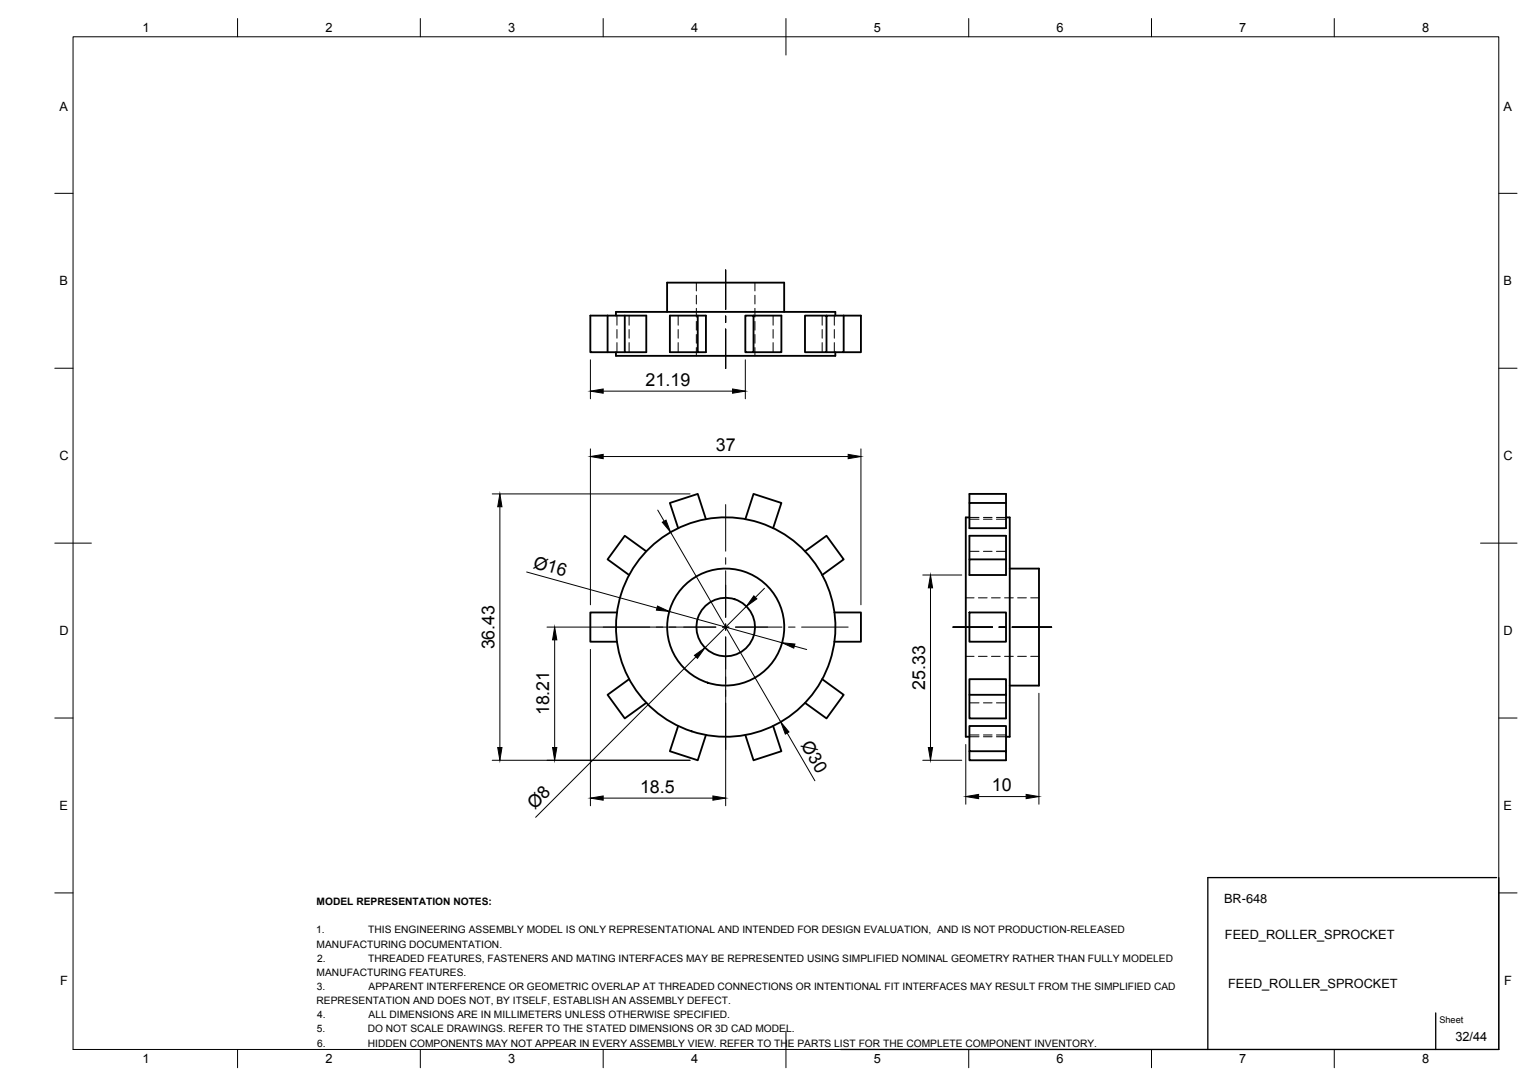
ISO-10303-21;
HEADER;
FILE_DESCRIPTION((''),'2;1');
FILE_NAME('FEED_ROLLER_SPROCKET.step','2026-10-01T22:05:39-07:00',(''),(''),'','','');
FILE_SCHEMA (('AUTOMOTIVE_DESIGN { 1 0 10303 214 3 1 1 }'));
ENDSEC;
DATA;
#10=MECHANICAL_DESIGN_GEOMETRIC_PRESENTATION_REPRESENTATION('',(#630),#24628);
#546=SHAPE_REPRESENTATION_RELATIONSHIP('SRR','None',#24819,#588) ;
#588=ADVANCED_BREP_SHAPE_REPRESENTATION('',(#669),#24609) ;
#630=STYLED_ITEM('',(#25030),#669) ;
#669=MANIFOLD_SOLID_BREP('FEED_ROLLER_SPROCKET',#13172) ;
#888=FACE_BOUND('',#4502,.T.) ;
#889=FACE_BOUND('',#4554,.T.) ;
#890=FACE_BOUND('',#4555,.T.) ;
#891=FACE_BOUND('',#4556,.T.) ;
#892=FACE_BOUND('',#4557,.T.) ;
#893=FACE_BOUND('',#4558,.T.) ;
#894=FACE_BOUND('',#4559,.T.) ;
#895=FACE_BOUND('',#4560,.T.) ;
#896=FACE_BOUND('',#4561,.T.) ;
#897=FACE_BOUND('',#4562,.T.) ;
#898=FACE_BOUND('',#4564,.T.) ;
#899=FACE_BOUND('',#4566,.T.) ;
#1562=LINE('',#23310,#2398) ;
#1563=LINE('',#23316,#2399) ;
#1564=LINE('',#23324,#2400) ;
#1565=LINE('',#23326,#2401) ;
#1566=LINE('',#23327,#2402) ;
#1567=LINE('',#23330,#2403) ;
#1568=LINE('',#23332,#2404) ;
#1569=LINE('',#23333,#2405) ;
#1570=LINE('',#23336,#2406) ;
#1571=LINE('',#23338,#2407) ;
#1572=LINE('',#23339,#2408) ;
#1573=LINE('',#23342,#2409) ;
#1574=LINE('',#23349,#2410) ;
#1575=LINE('',#23351,#2411) ;
#1576=LINE('',#23352,#2412) ;
#1577=LINE('',#23355,#2413) ;
#1578=LINE('',#23357,#2414) ;
#1579=LINE('',#23358,#2415) ;
#1580=LINE('',#23361,#2416) ;
#1581=LINE('',#23363,#2417) ;
#1582=LINE('',#23364,#2418) ;
#1583=LINE('',#23367,#2419) ;
#1584=LINE('',#23374,#2420) ;
#1585=LINE('',#23376,#2421) ;
#1586=LINE('',#23377,#2422) ;
#1587=LINE('',#23380,#2423) ;
#1588=LINE('',#23382,#2424) ;
#1589=LINE('',#23383,#2425) ;
#1590=LINE('',#23386,#2426) ;
#1591=LINE('',#23388,#2427) ;
#1592=LINE('',#23389,#2428) ;
#1593=LINE('',#23392,#2429) ;
#1594=LINE('',#23399,#2430) ;
#1595=LINE('',#23401,#2431) ;
#1596=LINE('',#23402,#2432) ;
#1597=LINE('',#23405,#2433) ;
#1598=LINE('',#23407,#2434) ;
#1599=LINE('',#23408,#2435) ;
#1600=LINE('',#23411,#2436) ;
#1601=LINE('',#23413,#2437) ;
#1602=LINE('',#23414,#2438) ;
#1603=LINE('',#23417,#2439) ;
#1604=LINE('',#23424,#2440) ;
#1605=LINE('',#23426,#2441) ;
#1606=LINE('',#23428,#2442) ;
#1607=LINE('',#23432,#2443) ;
#1608=LINE('',#23434,#2444) ;
#1609=LINE('',#23435,#2445) ;
#1610=LINE('',#23438,#2446) ;
#1611=LINE('',#23440,#2447) ;
#1612=LINE('',#23441,#2448) ;
#1613=LINE('',#23445,#2449) ;
#1614=LINE('',#23453,#2450) ;
#1615=LINE('',#23455,#2451) ;
#1616=LINE('',#23456,#2452) ;
#1617=LINE('',#23459,#2453) ;
#1618=LINE('',#23461,#2454) ;
#1619=LINE('',#23462,#2455) ;
#1620=LINE('',#23465,#2456) ;
#1621=LINE('',#23467,#2457) ;
#1622=LINE('',#23468,#2458) ;
#1623=LINE('',#23471,#2459) ;
#1624=LINE('',#23478,#2460) ;
#1625=LINE('',#23480,#2461) ;
#1626=LINE('',#23481,#2462) ;
#1627=LINE('',#23484,#2463) ;
#1628=LINE('',#23486,#2464) ;
#1629=LINE('',#23487,#2465) ;
#1630=LINE('',#23490,#2466) ;
#1631=LINE('',#23492,#2467) ;
#1632=LINE('',#23493,#2468) ;
#1633=LINE('',#23496,#2469) ;
#1634=LINE('',#23503,#2470) ;
#1635=LINE('',#23505,#2471) ;
#1636=LINE('',#23506,#2472) ;
#1637=LINE('',#23509,#2473) ;
#1638=LINE('',#23511,#2474) ;
#1639=LINE('',#23512,#2475) ;
#1640=LINE('',#23515,#2476) ;
#1641=LINE('',#23517,#2477) ;
#1642=LINE('',#23518,#2478) ;
#1643=LINE('',#23521,#2479) ;
#1644=LINE('',#23528,#2480) ;
#1645=LINE('',#23530,#2481) ;
#1646=LINE('',#23531,#2482) ;
#1647=LINE('',#23534,#2483) ;
#1648=LINE('',#23536,#2484) ;
#1649=LINE('',#23537,#2485) ;
#1650=LINE('',#23540,#2486) ;
#1651=LINE('',#23542,#2487) ;
#1652=LINE('',#23543,#2488) ;
#1653=LINE('',#23546,#2489) ;
#1654=LINE('',#23553,#2490) ;
#1655=LINE('',#23555,#2491) ;
#1656=LINE('',#23556,#2492) ;
#1657=LINE('',#23559,#2493) ;
#1658=LINE('',#23561,#2494) ;
#1659=LINE('',#23562,#2495) ;
#1660=LINE('',#23565,#2496) ;
#1661=LINE('',#23567,#2497) ;
#1662=LINE('',#23568,#2498) ;
#1663=LINE('',#23571,#2499) ;
#1664=LINE('',#23576,#2500) ;
#1665=LINE('',#23578,#2501) ;
#2398=VECTOR('',#18669,0.4) ;
#2399=VECTOR('',#18676,0.8) ;
#2400=VECTOR('',#18685,1.) ;
#2401=VECTOR('',#18686,1.) ;
#2402=VECTOR('',#18687,1.) ;
#2403=VECTOR('',#18690,1.) ;
#2404=VECTOR('',#18691,1.) ;
#2405=VECTOR('',#18692,1.) ;
#2406=VECTOR('',#18695,1.) ;
#2407=VECTOR('',#18696,1.) ;
#2408=VECTOR('',#18697,1.) ;
#2409=VECTOR('',#18702,1.) ;
#2410=VECTOR('',#18709,1.) ;
#2411=VECTOR('',#18710,1.) ;
#2412=VECTOR('',#18711,1.) ;
#2413=VECTOR('',#18714,1.) ;
#2414=VECTOR('',#18715,1.) ;
#2415=VECTOR('',#18716,1.) ;
#2416=VECTOR('',#18719,1.) ;
#2417=VECTOR('',#18720,1.) ;
#2418=VECTOR('',#18721,1.) ;
#2419=VECTOR('',#18726,1.) ;
#2420=VECTOR('',#18733,1.) ;
#2421=VECTOR('',#18734,1.) ;
#2422=VECTOR('',#18735,1.) ;
#2423=VECTOR('',#18738,1.) ;
#2424=VECTOR('',#18739,1.) ;
#2425=VECTOR('',#18740,1.) ;
#2426=VECTOR('',#18743,1.) ;
#2427=VECTOR('',#18744,1.) ;
#2428=VECTOR('',#18745,1.) ;
#2429=VECTOR('',#18750,1.) ;
#2430=VECTOR('',#18757,1.) ;
#2431=VECTOR('',#18758,1.) ;
#2432=VECTOR('',#18759,1.) ;
#2433=VECTOR('',#18762,1.) ;
#2434=VECTOR('',#18763,1.) ;
#2435=VECTOR('',#18764,1.) ;
#2436=VECTOR('',#18767,1.) ;
#2437=VECTOR('',#18768,1.) ;
#2438=VECTOR('',#18769,1.) ;
#2439=VECTOR('',#18774,1.) ;
#2440=VECTOR('',#18781,1.) ;
#2441=VECTOR('',#18782,1.) ;
#2442=VECTOR('',#18783,1.) ;
#2443=VECTOR('',#18788,1.) ;
#2444=VECTOR('',#18789,1.) ;
#2445=VECTOR('',#18790,1.) ;
#2446=VECTOR('',#18793,1.) ;
#2447=VECTOR('',#18794,1.) ;
#2448=VECTOR('',#18795,1.) ;
#2449=VECTOR('',#18800,1.) ;
#2450=VECTOR('',#18809,1.) ;
#2451=VECTOR('',#18810,1.) ;
#2452=VECTOR('',#18811,1.) ;
#2453=VECTOR('',#18814,1.) ;
#2454=VECTOR('',#18815,1.) ;
#2455=VECTOR('',#18816,1.) ;
#2456=VECTOR('',#18819,1.) ;
#2457=VECTOR('',#18820,1.) ;
#2458=VECTOR('',#18821,1.) ;
#2459=VECTOR('',#18826,1.) ;
#2460=VECTOR('',#18833,1.) ;
#2461=VECTOR('',#18834,1.) ;
#2462=VECTOR('',#18835,1.) ;
#2463=VECTOR('',#18838,1.) ;
#2464=VECTOR('',#18839,1.) ;
#2465=VECTOR('',#18840,1.) ;
#2466=VECTOR('',#18843,1.) ;
#2467=VECTOR('',#18844,1.) ;
#2468=VECTOR('',#18845,1.) ;
#2469=VECTOR('',#18850,1.) ;
#2470=VECTOR('',#18857,1.) ;
#2471=VECTOR('',#18858,1.) ;
#2472=VECTOR('',#18859,1.) ;
#2473=VECTOR('',#18862,1.) ;
#2474=VECTOR('',#18863,1.) ;
#2475=VECTOR('',#18864,1.) ;
#2476=VECTOR('',#18867,1.) ;
#2477=VECTOR('',#18868,1.) ;
#2478=VECTOR('',#18869,1.) ;
#2479=VECTOR('',#18874,1.) ;
#2480=VECTOR('',#18881,1.) ;
#2481=VECTOR('',#18882,1.) ;
#2482=VECTOR('',#18883,1.) ;
#2483=VECTOR('',#18886,1.) ;
#2484=VECTOR('',#18887,1.) ;
#2485=VECTOR('',#18888,1.) ;
#2486=VECTOR('',#18891,1.) ;
#2487=VECTOR('',#18892,1.) ;
#2488=VECTOR('',#18893,1.) ;
#2489=VECTOR('',#18898,1.) ;
#2490=VECTOR('',#18905,1.) ;
#2491=VECTOR('',#18906,1.) ;
#2492=VECTOR('',#18907,1.) ;
#2493=VECTOR('',#18910,1.) ;
#2494=VECTOR('',#18911,1.) ;
#2495=VECTOR('',#18912,1.) ;
#2496=VECTOR('',#18915,1.) ;
#2497=VECTOR('',#18916,1.) ;
#2498=VECTOR('',#18917,1.) ;
#2499=VECTOR('',#18922,1.) ;
#2500=VECTOR('',#18929,1.5) ;
#2501=VECTOR('',#18930,1.5) ;
#2900=CYLINDRICAL_SURFACE('',#15009,0.4) ;
#2901=CYLINDRICAL_SURFACE('',#15012,0.8) ;
#2902=CYLINDRICAL_SURFACE('',#15088,1.5) ;
#3530=FACE_OUTER_BOUND('',#4499,.T.) ;
#3531=FACE_OUTER_BOUND('',#4500,.T.) ;
#3532=FACE_OUTER_BOUND('',#4501,.T.) ;
#3533=FACE_OUTER_BOUND('',#4503,.T.) ;
#3534=FACE_OUTER_BOUND('',#4504,.T.) ;
#3535=FACE_OUTER_BOUND('',#4505,.T.) ;
#3536=FACE_OUTER_BOUND('',#4506,.T.) ;
#3537=FACE_OUTER_BOUND('',#4507,.T.) ;
#3538=FACE_OUTER_BOUND('',#4508,.T.) ;
#3539=FACE_OUTER_BOUND('',#4509,.T.) ;
#3540=FACE_OUTER_BOUND('',#4510,.T.) ;
#3541=FACE_OUTER_BOUND('',#4511,.T.) ;
#3542=FACE_OUTER_BOUND('',#4512,.T.) ;
#3543=FACE_OUTER_BOUND('',#4513,.T.) ;
#3544=FACE_OUTER_BOUND('',#4514,.T.) ;
#3545=FACE_OUTER_BOUND('',#4515,.T.) ;
#3546=FACE_OUTER_BOUND('',#4516,.T.) ;
#3547=FACE_OUTER_BOUND('',#4517,.T.) ;
#3548=FACE_OUTER_BOUND('',#4518,.T.) ;
#3549=FACE_OUTER_BOUND('',#4519,.T.) ;
#3550=FACE_OUTER_BOUND('',#4520,.T.) ;
#3551=FACE_OUTER_BOUND('',#4521,.T.) ;
#3552=FACE_OUTER_BOUND('',#4522,.T.) ;
#3553=FACE_OUTER_BOUND('',#4523,.T.) ;
#3554=FACE_OUTER_BOUND('',#4524,.T.) ;
#3555=FACE_OUTER_BOUND('',#4525,.T.) ;
#3556=FACE_OUTER_BOUND('',#4526,.T.) ;
#3557=FACE_OUTER_BOUND('',#4527,.T.) ;
#3558=FACE_OUTER_BOUND('',#4528,.T.) ;
#3559=FACE_OUTER_BOUND('',#4529,.T.) ;
#3560=FACE_OUTER_BOUND('',#4530,.T.) ;
#3561=FACE_OUTER_BOUND('',#4531,.T.) ;
#3562=FACE_OUTER_BOUND('',#4532,.T.) ;
#3563=FACE_OUTER_BOUND('',#4533,.T.) ;
#3564=FACE_OUTER_BOUND('',#4534,.T.) ;
#3565=FACE_OUTER_BOUND('',#4535,.T.) ;
#3566=FACE_OUTER_BOUND('',#4536,.T.) ;
#3567=FACE_OUTER_BOUND('',#4537,.T.) ;
#3568=FACE_OUTER_BOUND('',#4538,.T.) ;
#3569=FACE_OUTER_BOUND('',#4539,.T.) ;
#3570=FACE_OUTER_BOUND('',#4540,.T.) ;
#3571=FACE_OUTER_BOUND('',#4541,.T.) ;
#3572=FACE_OUTER_BOUND('',#4542,.T.) ;
#3573=FACE_OUTER_BOUND('',#4543,.T.) ;
#3574=FACE_OUTER_BOUND('',#4544,.T.) ;
#3575=FACE_OUTER_BOUND('',#4545,.T.) ;
#3576=FACE_OUTER_BOUND('',#4546,.T.) ;
#3577=FACE_OUTER_BOUND('',#4547,.T.) ;
#3578=FACE_OUTER_BOUND('',#4548,.T.) ;
#3579=FACE_OUTER_BOUND('',#4549,.T.) ;
#3580=FACE_OUTER_BOUND('',#4550,.T.) ;
#3581=FACE_OUTER_BOUND('',#4551,.T.) ;
#3582=FACE_OUTER_BOUND('',#4552,.T.) ;
#3583=FACE_OUTER_BOUND('',#4553,.T.) ;
#3584=FACE_OUTER_BOUND('',#4563,.T.) ;
#3585=FACE_OUTER_BOUND('',#4565,.T.) ;
#4499=EDGE_LOOP('',(#11147,#11148,#11149,#11150)) ;
#4500=EDGE_LOOP('',(#11151,#11152,#11153,#11154)) ;
#4501=EDGE_LOOP('',(#11155)) ;
#4502=EDGE_LOOP('',(#11156)) ;
#4503=EDGE_LOOP('',(#11157,#11158,#11159,#11160)) ;
#4504=EDGE_LOOP('',(#11161,#11162,#11163,#11164)) ;
#4505=EDGE_LOOP('',(#11165,#11166,#11167,#11168)) ;
#4506=EDGE_LOOP('',(#11169,#11170,#11171,#11172)) ;
#4507=EDGE_LOOP('',(#11173,#11174,#11175,#11176)) ;
#4508=EDGE_LOOP('',(#11177,#11178,#11179,#11180)) ;
#4509=EDGE_LOOP('',(#11181,#11182,#11183,#11184)) ;
#4510=EDGE_LOOP('',(#11185,#11186,#11187,#11188)) ;
#4511=EDGE_LOOP('',(#11189,#11190,#11191,#11192)) ;
#4512=EDGE_LOOP('',(#11193,#11194,#11195,#11196)) ;
#4513=EDGE_LOOP('',(#11197,#11198,#11199,#11200)) ;
#4514=EDGE_LOOP('',(#11201,#11202,#11203,#11204)) ;
#4515=EDGE_LOOP('',(#11205,#11206,#11207,#11208)) ;
#4516=EDGE_LOOP('',(#11209,#11210,#11211,#11212)) ;
#4517=EDGE_LOOP('',(#11213,#11214,#11215,#11216)) ;
#4518=EDGE_LOOP('',(#11217,#11218,#11219,#11220)) ;
#4519=EDGE_LOOP('',(#11221,#11222,#11223,#11224)) ;
#4520=EDGE_LOOP('',(#11225,#11226,#11227,#11228)) ;
#4521=EDGE_LOOP('',(#11229,#11230,#11231,#11232)) ;
#4522=EDGE_LOOP('',(#11233,#11234,#11235,#11236)) ;
#4523=EDGE_LOOP('',(#11237,#11238,#11239,#11240,#11241)) ;
#4524=EDGE_LOOP('',(#11242,#11243,#11244,#11245)) ;
#4525=EDGE_LOOP('',(#11246,#11247,#11248,#11249)) ;
#4526=EDGE_LOOP('',(#11250,#11251,#11252,#11253,#11254)) ;
#4527=EDGE_LOOP('',(#11255,#11256,#11257,#11258)) ;
#4528=EDGE_LOOP('',(#11259,#11260,#11261,#11262)) ;
#4529=EDGE_LOOP('',(#11263,#11264,#11265,#11266)) ;
#4530=EDGE_LOOP('',(#11267,#11268,#11269,#11270)) ;
#4531=EDGE_LOOP('',(#11271,#11272,#11273,#11274)) ;
#4532=EDGE_LOOP('',(#11275,#11276,#11277,#11278)) ;
#4533=EDGE_LOOP('',(#11279,#11280,#11281,#11282)) ;
#4534=EDGE_LOOP('',(#11283,#11284,#11285,#11286)) ;
#4535=EDGE_LOOP('',(#11287,#11288,#11289,#11290)) ;
#4536=EDGE_LOOP('',(#11291,#11292,#11293,#11294)) ;
#4537=EDGE_LOOP('',(#11295,#11296,#11297,#11298)) ;
#4538=EDGE_LOOP('',(#11299,#11300,#11301,#11302)) ;
#4539=EDGE_LOOP('',(#11303,#11304,#11305,#11306)) ;
#4540=EDGE_LOOP('',(#11307,#11308,#11309,#11310)) ;
#4541=EDGE_LOOP('',(#11311,#11312,#11313,#11314)) ;
#4542=EDGE_LOOP('',(#11315,#11316,#11317,#11318)) ;
#4543=EDGE_LOOP('',(#11319,#11320,#11321,#11322)) ;
#4544=EDGE_LOOP('',(#11323,#11324,#11325,#11326)) ;
#4545=EDGE_LOOP('',(#11327,#11328,#11329,#11330)) ;
#4546=EDGE_LOOP('',(#11331,#11332,#11333,#11334)) ;
#4547=EDGE_LOOP('',(#11335,#11336,#11337,#11338)) ;
#4548=EDGE_LOOP('',(#11339,#11340,#11341,#11342)) ;
#4549=EDGE_LOOP('',(#11343,#11344,#11345,#11346)) ;
#4550=EDGE_LOOP('',(#11347,#11348,#11349,#11350)) ;
#4551=EDGE_LOOP('',(#11351,#11352,#11353,#11354)) ;
#4552=EDGE_LOOP('',(#11355,#11356,#11357,#11358)) ;
#4553=EDGE_LOOP('',(#11359,#11360,#11361,#11362,#11363,#11364,#11365,#11366,
#11367,#11368,#11369,#11370)) ;
#4554=EDGE_LOOP('',(#11371,#11372,#11373,#11374)) ;
#4555=EDGE_LOOP('',(#11375,#11376,#11377,#11378)) ;
#4556=EDGE_LOOP('',(#11379,#11380,#11381,#11382)) ;
#4557=EDGE_LOOP('',(#11383,#11384,#11385,#11386)) ;
#4558=EDGE_LOOP('',(#11387,#11388,#11389,#11390)) ;
#4559=EDGE_LOOP('',(#11391,#11392,#11393,#11394)) ;
#4560=EDGE_LOOP('',(#11395,#11396,#11397,#11398)) ;
#4561=EDGE_LOOP('',(#11399,#11400,#11401,#11402)) ;
#4562=EDGE_LOOP('',(#11403,#11404,#11405,#11406)) ;
#4563=EDGE_LOOP('',(#11407)) ;
#4564=EDGE_LOOP('',(#11408)) ;
#4565=EDGE_LOOP('',(#11409)) ;
#4566=EDGE_LOOP('',(#11410)) ;
#5411=CIRCLE('',#15010,0.4) ;
#5412=CIRCLE('',#15011,0.4) ;
#5413=CIRCLE('',#15013,0.8) ;
#5414=CIRCLE('',#15014,0.8) ;
#5415=CIRCLE('',#15017,1.5) ;
#5416=CIRCLE('',#15021,1.5) ;
#5417=CIRCLE('',#15024,1.5) ;
#5418=CIRCLE('',#15028,1.5) ;
#5419=CIRCLE('',#15031,1.5) ;
#5420=CIRCLE('',#15035,1.5) ;
#5421=CIRCLE('',#15038,1.5) ;
#5422=CIRCLE('',#15042,1.5) ;
#5423=CIRCLE('',#15045,1.5) ;
#5424=CIRCLE('',#15046,1.5) ;
#5425=CIRCLE('',#15050,1.5) ;
#5426=CIRCLE('',#15051,1.5) ;
#5427=CIRCLE('',#15054,1.5) ;
#5428=CIRCLE('',#15058,1.5) ;
#5429=CIRCLE('',#15061,1.5) ;
#5430=CIRCLE('',#15065,1.5) ;
#5431=CIRCLE('',#15068,1.5) ;
#5432=CIRCLE('',#15072,1.5) ;
#5433=CIRCLE('',#15075,1.5) ;
#5434=CIRCLE('',#15079,1.5) ;
#5435=CIRCLE('',#15082,1.5) ;
#5436=CIRCLE('',#15086,1.5) ;
#5437=CIRCLE('',#15089,1.5) ;
#5438=CIRCLE('',#15090,1.5) ;
#6453=VERTEX_POINT('',#23307) ;
#6454=VERTEX_POINT('',#23309) ;
#6455=VERTEX_POINT('',#23313) ;
#6456=VERTEX_POINT('',#23315) ;
#6457=VERTEX_POINT('',#23320) ;
#6458=VERTEX_POINT('',#23321) ;
#6459=VERTEX_POINT('',#23323) ;
#6460=VERTEX_POINT('',#23325) ;
#6461=VERTEX_POINT('',#23329) ;
#6462=VERTEX_POINT('',#23331) ;
#6463=VERTEX_POINT('',#23335) ;
#6464=VERTEX_POINT('',#23337) ;
#6465=VERTEX_POINT('',#23345) ;
#6466=VERTEX_POINT('',#23346) ;
#6467=VERTEX_POINT('',#23348) ;
#6468=VERTEX_POINT('',#23350) ;
#6469=VERTEX_POINT('',#23354) ;
#6470=VERTEX_POINT('',#23356) ;
#6471=VERTEX_POINT('',#23360) ;
#6472=VERTEX_POINT('',#23362) ;
#6473=VERTEX_POINT('',#23370) ;
#6474=VERTEX_POINT('',#23371) ;
#6475=VERTEX_POINT('',#23373) ;
#6476=VERTEX_POINT('',#23375) ;
#6477=VERTEX_POINT('',#23379) ;
#6478=VERTEX_POINT('',#23381) ;
#6479=VERTEX_POINT('',#23385) ;
#6480=VERTEX_POINT('',#23387) ;
#6481=VERTEX_POINT('',#23395) ;
#6482=VERTEX_POINT('',#23396) ;
#6483=VERTEX_POINT('',#23398) ;
#6484=VERTEX_POINT('',#23400) ;
#6485=VERTEX_POINT('',#23404) ;
#6486=VERTEX_POINT('',#23406) ;
#6487=VERTEX_POINT('',#23410) ;
#6488=VERTEX_POINT('',#23412) ;
#6489=VERTEX_POINT('',#23420) ;
#6490=VERTEX_POINT('',#23421) ;
#6491=VERTEX_POINT('',#23423) ;
#6492=VERTEX_POINT('',#23425) ;
#6493=VERTEX_POINT('',#23427) ;
#6494=VERTEX_POINT('',#23431) ;
#6495=VERTEX_POINT('',#23433) ;
#6496=VERTEX_POINT('',#23437) ;
#6497=VERTEX_POINT('',#23439) ;
#6498=VERTEX_POINT('',#23443) ;
#6499=VERTEX_POINT('',#23449) ;
#6500=VERTEX_POINT('',#23450) ;
#6501=VERTEX_POINT('',#23452) ;
#6502=VERTEX_POINT('',#23454) ;
#6503=VERTEX_POINT('',#23458) ;
#6504=VERTEX_POINT('',#23460) ;
#6505=VERTEX_POINT('',#23464) ;
#6506=VERTEX_POINT('',#23466) ;
#6507=VERTEX_POINT('',#23474) ;
#6508=VERTEX_POINT('',#23475) ;
#6509=VERTEX_POINT('',#23477) ;
#6510=VERTEX_POINT('',#23479) ;
#6511=VERTEX_POINT('',#23483) ;
#6512=VERTEX_POINT('',#23485) ;
#6513=VERTEX_POINT('',#23489) ;
#6514=VERTEX_POINT('',#23491) ;
#6515=VERTEX_POINT('',#23499) ;
#6516=VERTEX_POINT('',#23500) ;
#6517=VERTEX_POINT('',#23502) ;
#6518=VERTEX_POINT('',#23504) ;
#6519=VERTEX_POINT('',#23508) ;
#6520=VERTEX_POINT('',#23510) ;
#6521=VERTEX_POINT('',#23514) ;
#6522=VERTEX_POINT('',#23516) ;
#6523=VERTEX_POINT('',#23524) ;
#6524=VERTEX_POINT('',#23525) ;
#6525=VERTEX_POINT('',#23527) ;
#6526=VERTEX_POINT('',#23529) ;
#6527=VERTEX_POINT('',#23533) ;
#6528=VERTEX_POINT('',#23535) ;
#6529=VERTEX_POINT('',#23539) ;
#6530=VERTEX_POINT('',#23541) ;
#6531=VERTEX_POINT('',#23549) ;
#6532=VERTEX_POINT('',#23550) ;
#6533=VERTEX_POINT('',#23552) ;
#6534=VERTEX_POINT('',#23554) ;
#6535=VERTEX_POINT('',#23558) ;
#6536=VERTEX_POINT('',#23560) ;
#6537=VERTEX_POINT('',#23564) ;
#6538=VERTEX_POINT('',#23566) ;
#6539=VERTEX_POINT('',#23574) ;
#6540=VERTEX_POINT('',#23577) ;
#8063=EDGE_CURVE('',#6453,#6453,#5411,.T.) ;
#8064=EDGE_CURVE('',#6453,#6454,#1562,.T.) ;
#8065=EDGE_CURVE('',#6454,#6454,#5412,.T.) ;
#8066=EDGE_CURVE('',#6455,#6455,#5413,.T.) ;
#8067=EDGE_CURVE('',#6455,#6456,#1563,.T.) ;
#8068=EDGE_CURVE('',#6456,#6456,#5414,.T.) ;
#8069=EDGE_CURVE('',#6457,#6458,#5415,.T.) ;
#8070=EDGE_CURVE('',#6459,#6457,#1564,.T.) ;
#8071=EDGE_CURVE('',#6460,#6459,#1565,.T.) ;
#8072=EDGE_CURVE('',#6458,#6460,#1566,.T.) ;
#8073=EDGE_CURVE('',#6461,#6457,#1567,.T.) ;
#8074=EDGE_CURVE('',#6461,#6462,#1568,.T.) ;
#8075=EDGE_CURVE('',#6462,#6459,#1569,.T.) ;
#8076=EDGE_CURVE('',#6458,#6463,#1570,.T.) ;
#8077=EDGE_CURVE('',#6460,#6464,#1571,.T.) ;
#8078=EDGE_CURVE('',#6464,#6463,#1572,.T.) ;
#8079=EDGE_CURVE('',#6463,#6461,#5416,.T.) ;
#8080=EDGE_CURVE('',#6464,#6462,#1573,.T.) ;
#8081=EDGE_CURVE('',#6465,#6466,#5417,.T.) ;
#8082=EDGE_CURVE('',#6467,#6465,#1574,.T.) ;
#8083=EDGE_CURVE('',#6468,#6467,#1575,.T.) ;
#8084=EDGE_CURVE('',#6466,#6468,#1576,.T.) ;
#8085=EDGE_CURVE('',#6469,#6465,#1577,.T.) ;
#8086=EDGE_CURVE('',#6469,#6470,#1578,.T.) ;
#8087=EDGE_CURVE('',#6470,#6467,#1579,.T.) ;
#8088=EDGE_CURVE('',#6466,#6471,#1580,.T.) ;
#8089=EDGE_CURVE('',#6468,#6472,#1581,.T.) ;
#8090=EDGE_CURVE('',#6472,#6471,#1582,.T.) ;
#8091=EDGE_CURVE('',#6471,#6469,#5418,.T.) ;
#8092=EDGE_CURVE('',#6472,#6470,#1583,.T.) ;
#8093=EDGE_CURVE('',#6473,#6474,#5419,.T.) ;
#8094=EDGE_CURVE('',#6475,#6473,#1584,.T.) ;
#8095=EDGE_CURVE('',#6476,#6475,#1585,.T.) ;
#8096=EDGE_CURVE('',#6474,#6476,#1586,.T.) ;
#8097=EDGE_CURVE('',#6477,#6473,#1587,.T.) ;
#8098=EDGE_CURVE('',#6477,#6478,#1588,.T.) ;
#8099=EDGE_CURVE('',#6478,#6475,#1589,.T.) ;
#8100=EDGE_CURVE('',#6474,#6479,#1590,.T.) ;
#8101=EDGE_CURVE('',#6476,#6480,#1591,.T.) ;
#8102=EDGE_CURVE('',#6480,#6479,#1592,.T.) ;
#8103=EDGE_CURVE('',#6479,#6477,#5420,.T.) ;
#8104=EDGE_CURVE('',#6480,#6478,#1593,.T.) ;
#8105=EDGE_CURVE('',#6481,#6482,#5421,.T.) ;
#8106=EDGE_CURVE('',#6483,#6481,#1594,.T.) ;
#8107=EDGE_CURVE('',#6484,#6483,#1595,.T.) ;
#8108=EDGE_CURVE('',#6482,#6484,#1596,.T.) ;
#8109=EDGE_CURVE('',#6485,#6481,#1597,.T.) ;
#8110=EDGE_CURVE('',#6485,#6486,#1598,.T.) ;
#8111=EDGE_CURVE('',#6486,#6483,#1599,.T.) ;
#8112=EDGE_CURVE('',#6482,#6487,#1600,.T.) ;
#8113=EDGE_CURVE('',#6484,#6488,#1601,.T.) ;
#8114=EDGE_CURVE('',#6488,#6487,#1602,.T.) ;
#8115=EDGE_CURVE('',#6487,#6485,#5422,.T.) ;
#8116=EDGE_CURVE('',#6488,#6486,#1603,.T.) ;
#8117=EDGE_CURVE('',#6489,#6490,#5423,.T.) ;
#8118=EDGE_CURVE('',#6491,#6489,#1604,.T.) ;
#8119=EDGE_CURVE('',#6492,#6491,#1605,.T.) ;
#8120=EDGE_CURVE('',#6493,#6492,#1606,.T.) ;
#8121=EDGE_CURVE('',#6490,#6493,#5424,.T.) ;
#8122=EDGE_CURVE('',#6494,#6489,#1607,.T.) ;
#8123=EDGE_CURVE('',#6494,#6495,#1608,.T.) ;
#8124=EDGE_CURVE('',#6495,#6491,#1609,.T.) ;
#8125=EDGE_CURVE('',#6493,#6496,#1610,.T.) ;
#8126=EDGE_CURVE('',#6492,#6497,#1611,.T.) ;
#8127=EDGE_CURVE('',#6497,#6496,#1612,.T.) ;
#8128=EDGE_CURVE('',#6496,#6498,#5425,.T.) ;
#8129=EDGE_CURVE('',#6497,#6495,#1613,.T.) ;
#8130=EDGE_CURVE('',#6498,#6494,#5426,.T.) ;
#8131=EDGE_CURVE('',#6499,#6500,#5427,.T.) ;
#8132=EDGE_CURVE('',#6501,#6499,#1614,.T.) ;
#8133=EDGE_CURVE('',#6502,#6501,#1615,.T.) ;
#8134=EDGE_CURVE('',#6500,#6502,#1616,.T.) ;
#8135=EDGE_CURVE('',#6503,#6499,#1617,.T.) ;
#8136=EDGE_CURVE('',#6503,#6504,#1618,.T.) ;
#8137=EDGE_CURVE('',#6504,#6501,#1619,.T.) ;
#8138=EDGE_CURVE('',#6500,#6505,#1620,.T.) ;
#8139=EDGE_CURVE('',#6502,#6506,#1621,.T.) ;
#8140=EDGE_CURVE('',#6506,#6505,#1622,.T.) ;
#8141=EDGE_CURVE('',#6505,#6503,#5428,.T.) ;
#8142=EDGE_CURVE('',#6506,#6504,#1623,.T.) ;
#8143=EDGE_CURVE('',#6507,#6508,#5429,.T.) ;
#8144=EDGE_CURVE('',#6509,#6507,#1624,.T.) ;
#8145=EDGE_CURVE('',#6510,#6509,#1625,.T.) ;
#8146=EDGE_CURVE('',#6508,#6510,#1626,.T.) ;
#8147=EDGE_CURVE('',#6511,#6507,#1627,.T.) ;
#8148=EDGE_CURVE('',#6511,#6512,#1628,.T.) ;
#8149=EDGE_CURVE('',#6512,#6509,#1629,.T.) ;
#8150=EDGE_CURVE('',#6508,#6513,#1630,.T.) ;
#8151=EDGE_CURVE('',#6510,#6514,#1631,.T.) ;
#8152=EDGE_CURVE('',#6514,#6513,#1632,.T.) ;
#8153=EDGE_CURVE('',#6513,#6511,#5430,.T.) ;
#8154=EDGE_CURVE('',#6514,#6512,#1633,.T.) ;
#8155=EDGE_CURVE('',#6515,#6516,#5431,.T.) ;
#8156=EDGE_CURVE('',#6517,#6515,#1634,.T.) ;
#8157=EDGE_CURVE('',#6518,#6517,#1635,.T.) ;
#8158=EDGE_CURVE('',#6516,#6518,#1636,.T.) ;
#8159=EDGE_CURVE('',#6519,#6515,#1637,.T.) ;
#8160=EDGE_CURVE('',#6519,#6520,#1638,.T.) ;
#8161=EDGE_CURVE('',#6520,#6517,#1639,.T.) ;
#8162=EDGE_CURVE('',#6516,#6521,#1640,.T.) ;
#8163=EDGE_CURVE('',#6518,#6522,#1641,.T.) ;
#8164=EDGE_CURVE('',#6522,#6521,#1642,.T.) ;
#8165=EDGE_CURVE('',#6521,#6519,#5432,.T.) ;
#8166=EDGE_CURVE('',#6522,#6520,#1643,.T.) ;
#8167=EDGE_CURVE('',#6523,#6524,#5433,.T.) ;
#8168=EDGE_CURVE('',#6525,#6523,#1644,.T.) ;
#8169=EDGE_CURVE('',#6526,#6525,#1645,.T.) ;
#8170=EDGE_CURVE('',#6524,#6526,#1646,.T.) ;
#8171=EDGE_CURVE('',#6527,#6523,#1647,.T.) ;
#8172=EDGE_CURVE('',#6527,#6528,#1648,.T.) ;
#8173=EDGE_CURVE('',#6528,#6525,#1649,.T.) ;
#8174=EDGE_CURVE('',#6524,#6529,#1650,.T.) ;
#8175=EDGE_CURVE('',#6526,#6530,#1651,.T.) ;
#8176=EDGE_CURVE('',#6530,#6529,#1652,.T.) ;
#8177=EDGE_CURVE('',#6529,#6527,#5434,.T.) ;
#8178=EDGE_CURVE('',#6530,#6528,#1653,.T.) ;
#8179=EDGE_CURVE('',#6531,#6532,#5435,.T.) ;
#8180=EDGE_CURVE('',#6533,#6531,#1654,.T.) ;
#8181=EDGE_CURVE('',#6534,#6533,#1655,.T.) ;
#8182=EDGE_CURVE('',#6532,#6534,#1656,.T.) ;
#8183=EDGE_CURVE('',#6535,#6531,#1657,.T.) ;
#8184=EDGE_CURVE('',#6535,#6536,#1658,.T.) ;
#8185=EDGE_CURVE('',#6536,#6533,#1659,.T.) ;
#8186=EDGE_CURVE('',#6532,#6537,#1660,.T.) ;
#8187=EDGE_CURVE('',#6534,#6538,#1661,.T.) ;
#8188=EDGE_CURVE('',#6538,#6537,#1662,.T.) ;
#8189=EDGE_CURVE('',#6537,#6535,#5436,.T.) ;
#8190=EDGE_CURVE('',#6538,#6536,#1663,.T.) ;
#8191=EDGE_CURVE('',#6539,#6539,#5437,.T.) ;
#8192=EDGE_CURVE('',#6539,#6498,#1664,.T.) ;
#8193=EDGE_CURVE('',#6490,#6540,#1665,.T.) ;
#8194=EDGE_CURVE('',#6540,#6540,#5438,.T.) ;
#11147=ORIENTED_EDGE('',*,*,#8063,.F.) ;
#11148=ORIENTED_EDGE('',*,*,#8064,.T.) ;
#11149=ORIENTED_EDGE('',*,*,#8065,.F.) ;
#11150=ORIENTED_EDGE('',*,*,#8064,.F.) ;
#11151=ORIENTED_EDGE('',*,*,#8066,.F.) ;
#11152=ORIENTED_EDGE('',*,*,#8067,.T.) ;
#11153=ORIENTED_EDGE('',*,*,#8068,.F.) ;
#11154=ORIENTED_EDGE('',*,*,#8067,.F.) ;
#11155=ORIENTED_EDGE('',*,*,#8068,.T.) ;
#11156=ORIENTED_EDGE('',*,*,#8063,.T.) ;
#11157=ORIENTED_EDGE('',*,*,#8069,.F.) ;
#11158=ORIENTED_EDGE('',*,*,#8070,.F.) ;
#11159=ORIENTED_EDGE('',*,*,#8071,.F.) ;
#11160=ORIENTED_EDGE('',*,*,#8072,.F.) ;
#11161=ORIENTED_EDGE('',*,*,#8073,.F.) ;
#11162=ORIENTED_EDGE('',*,*,#8074,.T.) ;
#11163=ORIENTED_EDGE('',*,*,#8075,.T.) ;
#11164=ORIENTED_EDGE('',*,*,#8070,.T.) ;
#11165=ORIENTED_EDGE('',*,*,#8076,.F.) ;
#11166=ORIENTED_EDGE('',*,*,#8072,.T.) ;
#11167=ORIENTED_EDGE('',*,*,#8077,.T.) ;
#11168=ORIENTED_EDGE('',*,*,#8078,.T.) ;
#11169=ORIENTED_EDGE('',*,*,#8079,.F.) ;
#11170=ORIENTED_EDGE('',*,*,#8078,.F.) ;
#11171=ORIENTED_EDGE('',*,*,#8080,.T.) ;
#11172=ORIENTED_EDGE('',*,*,#8074,.F.) ;
#11173=ORIENTED_EDGE('',*,*,#8071,.T.) ;
#11174=ORIENTED_EDGE('',*,*,#8075,.F.) ;
#11175=ORIENTED_EDGE('',*,*,#8080,.F.) ;
#11176=ORIENTED_EDGE('',*,*,#8077,.F.) ;
#11177=ORIENTED_EDGE('',*,*,#8081,.F.) ;
#11178=ORIENTED_EDGE('',*,*,#8082,.F.) ;
#11179=ORIENTED_EDGE('',*,*,#8083,.F.) ;
#11180=ORIENTED_EDGE('',*,*,#8084,.F.) ;
#11181=ORIENTED_EDGE('',*,*,#8085,.F.) ;
#11182=ORIENTED_EDGE('',*,*,#8086,.T.) ;
#11183=ORIENTED_EDGE('',*,*,#8087,.T.) ;
#11184=ORIENTED_EDGE('',*,*,#8082,.T.) ;
#11185=ORIENTED_EDGE('',*,*,#8088,.F.) ;
#11186=ORIENTED_EDGE('',*,*,#8084,.T.) ;
#11187=ORIENTED_EDGE('',*,*,#8089,.T.) ;
#11188=ORIENTED_EDGE('',*,*,#8090,.T.) ;
#11189=ORIENTED_EDGE('',*,*,#8091,.F.) ;
#11190=ORIENTED_EDGE('',*,*,#8090,.F.) ;
#11191=ORIENTED_EDGE('',*,*,#8092,.T.) ;
#11192=ORIENTED_EDGE('',*,*,#8086,.F.) ;
#11193=ORIENTED_EDGE('',*,*,#8083,.T.) ;
#11194=ORIENTED_EDGE('',*,*,#8087,.F.) ;
#11195=ORIENTED_EDGE('',*,*,#8092,.F.) ;
#11196=ORIENTED_EDGE('',*,*,#8089,.F.) ;
#11197=ORIENTED_EDGE('',*,*,#8093,.F.) ;
#11198=ORIENTED_EDGE('',*,*,#8094,.F.) ;
#11199=ORIENTED_EDGE('',*,*,#8095,.F.) ;
#11200=ORIENTED_EDGE('',*,*,#8096,.F.) ;
#11201=ORIENTED_EDGE('',*,*,#8097,.F.) ;
#11202=ORIENTED_EDGE('',*,*,#8098,.T.) ;
#11203=ORIENTED_EDGE('',*,*,#8099,.T.) ;
#11204=ORIENTED_EDGE('',*,*,#8094,.T.) ;
#11205=ORIENTED_EDGE('',*,*,#8100,.F.) ;
#11206=ORIENTED_EDGE('',*,*,#8096,.T.) ;
#11207=ORIENTED_EDGE('',*,*,#8101,.T.) ;
#11208=ORIENTED_EDGE('',*,*,#8102,.T.) ;
#11209=ORIENTED_EDGE('',*,*,#8103,.F.) ;
#11210=ORIENTED_EDGE('',*,*,#8102,.F.) ;
#11211=ORIENTED_EDGE('',*,*,#8104,.T.) ;
#11212=ORIENTED_EDGE('',*,*,#8098,.F.) ;
#11213=ORIENTED_EDGE('',*,*,#8095,.T.) ;
#11214=ORIENTED_EDGE('',*,*,#8099,.F.) ;
#11215=ORIENTED_EDGE('',*,*,#8104,.F.) ;
#11216=ORIENTED_EDGE('',*,*,#8101,.F.) ;
#11217=ORIENTED_EDGE('',*,*,#8105,.F.) ;
#11218=ORIENTED_EDGE('',*,*,#8106,.F.) ;
#11219=ORIENTED_EDGE('',*,*,#8107,.F.) ;
#11220=ORIENTED_EDGE('',*,*,#8108,.F.) ;
#11221=ORIENTED_EDGE('',*,*,#8109,.F.) ;
#11222=ORIENTED_EDGE('',*,*,#8110,.T.) ;
#11223=ORIENTED_EDGE('',*,*,#8111,.T.) ;
#11224=ORIENTED_EDGE('',*,*,#8106,.T.) ;
#11225=ORIENTED_EDGE('',*,*,#8112,.F.) ;
#11226=ORIENTED_EDGE('',*,*,#8108,.T.) ;
#11227=ORIENTED_EDGE('',*,*,#8113,.T.) ;
#11228=ORIENTED_EDGE('',*,*,#8114,.T.) ;
#11229=ORIENTED_EDGE('',*,*,#8115,.F.) ;
#11230=ORIENTED_EDGE('',*,*,#8114,.F.) ;
#11231=ORIENTED_EDGE('',*,*,#8116,.T.) ;
#11232=ORIENTED_EDGE('',*,*,#8110,.F.) ;
#11233=ORIENTED_EDGE('',*,*,#8107,.T.) ;
#11234=ORIENTED_EDGE('',*,*,#8111,.F.) ;
#11235=ORIENTED_EDGE('',*,*,#8116,.F.) ;
#11236=ORIENTED_EDGE('',*,*,#8113,.F.) ;
#11237=ORIENTED_EDGE('',*,*,#8117,.F.) ;
#11238=ORIENTED_EDGE('',*,*,#8118,.F.) ;
#11239=ORIENTED_EDGE('',*,*,#8119,.F.) ;
#11240=ORIENTED_EDGE('',*,*,#8120,.F.) ;
#11241=ORIENTED_EDGE('',*,*,#8121,.F.) ;
#11242=ORIENTED_EDGE('',*,*,#8122,.F.) ;
#11243=ORIENTED_EDGE('',*,*,#8123,.T.) ;
#11244=ORIENTED_EDGE('',*,*,#8124,.T.) ;
#11245=ORIENTED_EDGE('',*,*,#8118,.T.) ;
#11246=ORIENTED_EDGE('',*,*,#8125,.F.) ;
#11247=ORIENTED_EDGE('',*,*,#8120,.T.) ;
#11248=ORIENTED_EDGE('',*,*,#8126,.T.) ;
#11249=ORIENTED_EDGE('',*,*,#8127,.T.) ;
#11250=ORIENTED_EDGE('',*,*,#8128,.F.) ;
#11251=ORIENTED_EDGE('',*,*,#8127,.F.) ;
#11252=ORIENTED_EDGE('',*,*,#8129,.T.) ;
#11253=ORIENTED_EDGE('',*,*,#8123,.F.) ;
#11254=ORIENTED_EDGE('',*,*,#8130,.F.) ;
#11255=ORIENTED_EDGE('',*,*,#8119,.T.) ;
#11256=ORIENTED_EDGE('',*,*,#8124,.F.) ;
#11257=ORIENTED_EDGE('',*,*,#8129,.F.) ;
#11258=ORIENTED_EDGE('',*,*,#8126,.F.) ;
#11259=ORIENTED_EDGE('',*,*,#8131,.F.) ;
#11260=ORIENTED_EDGE('',*,*,#8132,.F.) ;
#11261=ORIENTED_EDGE('',*,*,#8133,.F.) ;
#11262=ORIENTED_EDGE('',*,*,#8134,.F.) ;
#11263=ORIENTED_EDGE('',*,*,#8135,.F.) ;
#11264=ORIENTED_EDGE('',*,*,#8136,.T.) ;
#11265=ORIENTED_EDGE('',*,*,#8137,.T.) ;
#11266=ORIENTED_EDGE('',*,*,#8132,.T.) ;
#11267=ORIENTED_EDGE('',*,*,#8138,.F.) ;
#11268=ORIENTED_EDGE('',*,*,#8134,.T.) ;
#11269=ORIENTED_EDGE('',*,*,#8139,.T.) ;
#11270=ORIENTED_EDGE('',*,*,#8140,.T.) ;
#11271=ORIENTED_EDGE('',*,*,#8141,.F.) ;
#11272=ORIENTED_EDGE('',*,*,#8140,.F.) ;
#11273=ORIENTED_EDGE('',*,*,#8142,.T.) ;
#11274=ORIENTED_EDGE('',*,*,#8136,.F.) ;
#11275=ORIENTED_EDGE('',*,*,#8133,.T.) ;
#11276=ORIENTED_EDGE('',*,*,#8137,.F.) ;
#11277=ORIENTED_EDGE('',*,*,#8142,.F.) ;
#11278=ORIENTED_EDGE('',*,*,#8139,.F.) ;
#11279=ORIENTED_EDGE('',*,*,#8143,.F.) ;
#11280=ORIENTED_EDGE('',*,*,#8144,.F.) ;
#11281=ORIENTED_EDGE('',*,*,#8145,.F.) ;
#11282=ORIENTED_EDGE('',*,*,#8146,.F.) ;
#11283=ORIENTED_EDGE('',*,*,#8147,.F.) ;
#11284=ORIENTED_EDGE('',*,*,#8148,.T.) ;
#11285=ORIENTED_EDGE('',*,*,#8149,.T.) ;
#11286=ORIENTED_EDGE('',*,*,#8144,.T.) ;
#11287=ORIENTED_EDGE('',*,*,#8150,.F.) ;
#11288=ORIENTED_EDGE('',*,*,#8146,.T.) ;
#11289=ORIENTED_EDGE('',*,*,#8151,.T.) ;
#11290=ORIENTED_EDGE('',*,*,#8152,.T.) ;
#11291=ORIENTED_EDGE('',*,*,#8153,.F.) ;
#11292=ORIENTED_EDGE('',*,*,#8152,.F.) ;
#11293=ORIENTED_EDGE('',*,*,#8154,.T.) ;
#11294=ORIENTED_EDGE('',*,*,#8148,.F.) ;
#11295=ORIENTED_EDGE('',*,*,#8145,.T.) ;
#11296=ORIENTED_EDGE('',*,*,#8149,.F.) ;
#11297=ORIENTED_EDGE('',*,*,#8154,.F.) ;
#11298=ORIENTED_EDGE('',*,*,#8151,.F.) ;
#11299=ORIENTED_EDGE('',*,*,#8155,.F.) ;
#11300=ORIENTED_EDGE('',*,*,#8156,.F.) ;
#11301=ORIENTED_EDGE('',*,*,#8157,.F.) ;
#11302=ORIENTED_EDGE('',*,*,#8158,.F.) ;
#11303=ORIENTED_EDGE('',*,*,#8159,.F.) ;
#11304=ORIENTED_EDGE('',*,*,#8160,.T.) ;
#11305=ORIENTED_EDGE('',*,*,#8161,.T.) ;
#11306=ORIENTED_EDGE('',*,*,#8156,.T.) ;
#11307=ORIENTED_EDGE('',*,*,#8162,.F.) ;
#11308=ORIENTED_EDGE('',*,*,#8158,.T.) ;
#11309=ORIENTED_EDGE('',*,*,#8163,.T.) ;
#11310=ORIENTED_EDGE('',*,*,#8164,.T.) ;
#11311=ORIENTED_EDGE('',*,*,#8165,.F.) ;
#11312=ORIENTED_EDGE('',*,*,#8164,.F.) ;
#11313=ORIENTED_EDGE('',*,*,#8166,.T.) ;
#11314=ORIENTED_EDGE('',*,*,#8160,.F.) ;
#11315=ORIENTED_EDGE('',*,*,#8157,.T.) ;
#11316=ORIENTED_EDGE('',*,*,#8161,.F.) ;
#11317=ORIENTED_EDGE('',*,*,#8166,.F.) ;
#11318=ORIENTED_EDGE('',*,*,#8163,.F.) ;
#11319=ORIENTED_EDGE('',*,*,#8167,.F.) ;
#11320=ORIENTED_EDGE('',*,*,#8168,.F.) ;
#11321=ORIENTED_EDGE('',*,*,#8169,.F.) ;
#11322=ORIENTED_EDGE('',*,*,#8170,.F.) ;
#11323=ORIENTED_EDGE('',*,*,#8171,.F.) ;
#11324=ORIENTED_EDGE('',*,*,#8172,.T.) ;
#11325=ORIENTED_EDGE('',*,*,#8173,.T.) ;
#11326=ORIENTED_EDGE('',*,*,#8168,.T.) ;
#11327=ORIENTED_EDGE('',*,*,#8174,.F.) ;
#11328=ORIENTED_EDGE('',*,*,#8170,.T.) ;
#11329=ORIENTED_EDGE('',*,*,#8175,.T.) ;
#11330=ORIENTED_EDGE('',*,*,#8176,.T.) ;
#11331=ORIENTED_EDGE('',*,*,#8177,.F.) ;
#11332=ORIENTED_EDGE('',*,*,#8176,.F.) ;
#11333=ORIENTED_EDGE('',*,*,#8178,.T.) ;
#11334=ORIENTED_EDGE('',*,*,#8172,.F.) ;
#11335=ORIENTED_EDGE('',*,*,#8169,.T.) ;
#11336=ORIENTED_EDGE('',*,*,#8173,.F.) ;
#11337=ORIENTED_EDGE('',*,*,#8178,.F.) ;
#11338=ORIENTED_EDGE('',*,*,#8175,.F.) ;
#11339=ORIENTED_EDGE('',*,*,#8179,.F.) ;
#11340=ORIENTED_EDGE('',*,*,#8180,.F.) ;
#11341=ORIENTED_EDGE('',*,*,#8181,.F.) ;
#11342=ORIENTED_EDGE('',*,*,#8182,.F.) ;
#11343=ORIENTED_EDGE('',*,*,#8183,.F.) ;
#11344=ORIENTED_EDGE('',*,*,#8184,.T.) ;
#11345=ORIENTED_EDGE('',*,*,#8185,.T.) ;
#11346=ORIENTED_EDGE('',*,*,#8180,.T.) ;
#11347=ORIENTED_EDGE('',*,*,#8186,.F.) ;
#11348=ORIENTED_EDGE('',*,*,#8182,.T.) ;
#11349=ORIENTED_EDGE('',*,*,#8187,.T.) ;
#11350=ORIENTED_EDGE('',*,*,#8188,.T.) ;
#11351=ORIENTED_EDGE('',*,*,#8189,.F.) ;
#11352=ORIENTED_EDGE('',*,*,#8188,.F.) ;
#11353=ORIENTED_EDGE('',*,*,#8190,.T.) ;
#11354=ORIENTED_EDGE('',*,*,#8184,.F.) ;
#11355=ORIENTED_EDGE('',*,*,#8181,.T.) ;
#11356=ORIENTED_EDGE('',*,*,#8185,.F.) ;
#11357=ORIENTED_EDGE('',*,*,#8190,.F.) ;
#11358=ORIENTED_EDGE('',*,*,#8187,.F.) ;
#11359=ORIENTED_EDGE('',*,*,#8191,.F.) ;
#11360=ORIENTED_EDGE('',*,*,#8192,.T.) ;
#11361=ORIENTED_EDGE('',*,*,#8130,.T.) ;
#11362=ORIENTED_EDGE('',*,*,#8122,.T.) ;
#11363=ORIENTED_EDGE('',*,*,#8117,.T.) ;
#11364=ORIENTED_EDGE('',*,*,#8193,.T.) ;
#11365=ORIENTED_EDGE('',*,*,#8194,.F.) ;
#11366=ORIENTED_EDGE('',*,*,#8193,.F.) ;
#11367=ORIENTED_EDGE('',*,*,#8121,.T.) ;
#11368=ORIENTED_EDGE('',*,*,#8125,.T.) ;
#11369=ORIENTED_EDGE('',*,*,#8128,.T.) ;
#11370=ORIENTED_EDGE('',*,*,#8192,.F.) ;
#11371=ORIENTED_EDGE('',*,*,#8073,.T.) ;
#11372=ORIENTED_EDGE('',*,*,#8069,.T.) ;
#11373=ORIENTED_EDGE('',*,*,#8076,.T.) ;
#11374=ORIENTED_EDGE('',*,*,#8079,.T.) ;
#11375=ORIENTED_EDGE('',*,*,#8085,.T.) ;
#11376=ORIENTED_EDGE('',*,*,#8081,.T.) ;
#11377=ORIENTED_EDGE('',*,*,#8088,.T.) ;
#11378=ORIENTED_EDGE('',*,*,#8091,.T.) ;
#11379=ORIENTED_EDGE('',*,*,#8097,.T.) ;
#11380=ORIENTED_EDGE('',*,*,#8093,.T.) ;
#11381=ORIENTED_EDGE('',*,*,#8100,.T.) ;
#11382=ORIENTED_EDGE('',*,*,#8103,.T.) ;
#11383=ORIENTED_EDGE('',*,*,#8109,.T.) ;
#11384=ORIENTED_EDGE('',*,*,#8105,.T.) ;
#11385=ORIENTED_EDGE('',*,*,#8112,.T.) ;
#11386=ORIENTED_EDGE('',*,*,#8115,.T.) ;
#11387=ORIENTED_EDGE('',*,*,#8135,.T.) ;
#11388=ORIENTED_EDGE('',*,*,#8131,.T.) ;
#11389=ORIENTED_EDGE('',*,*,#8138,.T.) ;
#11390=ORIENTED_EDGE('',*,*,#8141,.T.) ;
#11391=ORIENTED_EDGE('',*,*,#8147,.T.) ;
#11392=ORIENTED_EDGE('',*,*,#8143,.T.) ;
#11393=ORIENTED_EDGE('',*,*,#8150,.T.) ;
#11394=ORIENTED_EDGE('',*,*,#8153,.T.) ;
#11395=ORIENTED_EDGE('',*,*,#8159,.T.) ;
#11396=ORIENTED_EDGE('',*,*,#8155,.T.) ;
#11397=ORIENTED_EDGE('',*,*,#8162,.T.) ;
#11398=ORIENTED_EDGE('',*,*,#8165,.T.) ;
#11399=ORIENTED_EDGE('',*,*,#8171,.T.) ;
#11400=ORIENTED_EDGE('',*,*,#8167,.T.) ;
#11401=ORIENTED_EDGE('',*,*,#8174,.T.) ;
#11402=ORIENTED_EDGE('',*,*,#8177,.T.) ;
#11403=ORIENTED_EDGE('',*,*,#8183,.T.) ;
#11404=ORIENTED_EDGE('',*,*,#8179,.T.) ;
#11405=ORIENTED_EDGE('',*,*,#8186,.T.) ;
#11406=ORIENTED_EDGE('',*,*,#8189,.T.) ;
#11407=ORIENTED_EDGE('',*,*,#8194,.T.) ;
#11408=ORIENTED_EDGE('',*,*,#8066,.T.) ;
#11409=ORIENTED_EDGE('',*,*,#8191,.T.) ;
#11410=ORIENTED_EDGE('',*,*,#8065,.T.) ;
#12215=PLANE('',#15015) ;
#12216=PLANE('',#15016) ;
#12217=PLANE('',#15018) ;
#12218=PLANE('',#15019) ;
#12219=PLANE('',#15020) ;
#12220=PLANE('',#15022) ;
#12221=PLANE('',#15023) ;
#12222=PLANE('',#15025) ;
#12223=PLANE('',#15026) ;
#12224=PLANE('',#15027) ;
#12225=PLANE('',#15029) ;
#12226=PLANE('',#15030) ;
#12227=PLANE('',#15032) ;
#12228=PLANE('',#15033) ;
#12229=PLANE('',#15034) ;
#12230=PLANE('',#15036) ;
#12231=PLANE('',#15037) ;
#12232=PLANE('',#15039) ;
#12233=PLANE('',#15040) ;
#12234=PLANE('',#15041) ;
#12235=PLANE('',#15043) ;
#12236=PLANE('',#15044) ;
#12237=PLANE('',#15047) ;
#12238=PLANE('',#15048) ;
#12239=PLANE('',#15049) ;
#12240=PLANE('',#15052) ;
#12241=PLANE('',#15053) ;
#12242=PLANE('',#15055) ;
#12243=PLANE('',#15056) ;
#12244=PLANE('',#15057) ;
#12245=PLANE('',#15059) ;
#12246=PLANE('',#15060) ;
#12247=PLANE('',#15062) ;
#12248=PLANE('',#15063) ;
#12249=PLANE('',#15064) ;
#12250=PLANE('',#15066) ;
#12251=PLANE('',#15067) ;
#12252=PLANE('',#15069) ;
#12253=PLANE('',#15070) ;
#12254=PLANE('',#15071) ;
#12255=PLANE('',#15073) ;
#12256=PLANE('',#15074) ;
#12257=PLANE('',#15076) ;
#12258=PLANE('',#15077) ;
#12259=PLANE('',#15078) ;
#12260=PLANE('',#15080) ;
#12261=PLANE('',#15081) ;
#12262=PLANE('',#15083) ;
#12263=PLANE('',#15084) ;
#12264=PLANE('',#15085) ;
#12265=PLANE('',#15087) ;
#12266=PLANE('',#15091) ;
#12267=PLANE('',#15092) ;
#12925=ADVANCED_FACE('',(#3530),#2900,.F.) ;
#12926=ADVANCED_FACE('',(#3531),#2901,.T.) ;
#12927=ADVANCED_FACE('',(#3532,#888),#12215,.T.) ;
#12928=ADVANCED_FACE('',(#3533),#12216,.F.) ;
#12929=ADVANCED_FACE('',(#3534),#12217,.F.) ;
#12930=ADVANCED_FACE('',(#3535),#12218,.T.) ;
#12931=ADVANCED_FACE('',(#3536),#12219,.F.) ;
#12932=ADVANCED_FACE('',(#3537),#12220,.F.) ;
#12933=ADVANCED_FACE('',(#3538),#12221,.F.) ;
#12934=ADVANCED_FACE('',(#3539),#12222,.F.) ;
#12935=ADVANCED_FACE('',(#3540),#12223,.T.) ;
#12936=ADVANCED_FACE('',(#3541),#12224,.F.) ;
#12937=ADVANCED_FACE('',(#3542),#12225,.F.) ;
#12938=ADVANCED_FACE('',(#3543),#12226,.F.) ;
#12939=ADVANCED_FACE('',(#3544),#12227,.F.) ;
#12940=ADVANCED_FACE('',(#3545),#12228,.T.) ;
#12941=ADVANCED_FACE('',(#3546),#12229,.F.) ;
#12942=ADVANCED_FACE('',(#3547),#12230,.F.) ;
#12943=ADVANCED_FACE('',(#3548),#12231,.F.) ;
#12944=ADVANCED_FACE('',(#3549),#12232,.F.) ;
#12945=ADVANCED_FACE('',(#3550),#12233,.T.) ;
#12946=ADVANCED_FACE('',(#3551),#12234,.F.) ;
#12947=ADVANCED_FACE('',(#3552),#12235,.F.) ;
#12948=ADVANCED_FACE('',(#3553),#12236,.F.) ;
#12949=ADVANCED_FACE('',(#3554),#12237,.F.) ;
#12950=ADVANCED_FACE('',(#3555),#12238,.T.) ;
#12951=ADVANCED_FACE('',(#3556),#12239,.F.) ;
#12952=ADVANCED_FACE('',(#3557),#12240,.F.) ;
#12953=ADVANCED_FACE('',(#3558),#12241,.F.) ;
#12954=ADVANCED_FACE('',(#3559),#12242,.F.) ;
#12955=ADVANCED_FACE('',(#3560),#12243,.T.) ;
#12956=ADVANCED_FACE('',(#3561),#12244,.F.) ;
#12957=ADVANCED_FACE('',(#3562),#12245,.F.) ;
#12958=ADVANCED_FACE('',(#3563),#12246,.F.) ;
#12959=ADVANCED_FACE('',(#3564),#12247,.F.) ;
#12960=ADVANCED_FACE('',(#3565),#12248,.T.) ;
#12961=ADVANCED_FACE('',(#3566),#12249,.F.) ;
#12962=ADVANCED_FACE('',(#3567),#12250,.F.) ;
#12963=ADVANCED_FACE('',(#3568),#12251,.F.) ;
#12964=ADVANCED_FACE('',(#3569),#12252,.F.) ;
#12965=ADVANCED_FACE('',(#3570),#12253,.T.) ;
#12966=ADVANCED_FACE('',(#3571),#12254,.F.) ;
#12967=ADVANCED_FACE('',(#3572),#12255,.F.) ;
#12968=ADVANCED_FACE('',(#3573),#12256,.F.) ;
#12969=ADVANCED_FACE('',(#3574),#12257,.F.) ;
#12970=ADVANCED_FACE('',(#3575),#12258,.T.) ;
#12971=ADVANCED_FACE('',(#3576),#12259,.F.) ;
#12972=ADVANCED_FACE('',(#3577),#12260,.F.) ;
#12973=ADVANCED_FACE('',(#3578),#12261,.F.) ;
#12974=ADVANCED_FACE('',(#3579),#12262,.F.) ;
#12975=ADVANCED_FACE('',(#3580),#12263,.T.) ;
#12976=ADVANCED_FACE('',(#3581),#12264,.F.) ;
#12977=ADVANCED_FACE('',(#3582),#12265,.F.) ;
#12978=ADVANCED_FACE('',(#3583,#889,#890,#891,#892,#893,#894,#895,#896,
#897),#2902,.T.) ;
#12979=ADVANCED_FACE('',(#3584,#898),#12266,.T.) ;
#12980=ADVANCED_FACE('',(#3585,#899),#12267,.T.) ;
#13172=CLOSED_SHELL('',(#12925,#12926,#12927,#12928,#12929,#12930,#12931,
#12932,#12933,#12934,#12935,#12936,#12937,#12938,#12939,#12940,#12941,#12942,
#12943,#12944,#12945,#12946,#12947,#12948,#12949,#12950,#12951,#12952,#12953,
#12954,#12955,#12956,#12957,#12958,#12959,#12960,#12961,#12962,#12963,#12964,
#12965,#12966,#12967,#12968,#12969,#12970,#12971,#12972,#12973,#12974,#12975,
#12976,#12977,#12978,#12979,#12980)) ;
#15008=AXIS2_PLACEMENT_3D('',#23305,#18663,#18664) ;
#15009=AXIS2_PLACEMENT_3D('',#23306,#18665,#18666) ;
#15010=AXIS2_PLACEMENT_3D('',#23308,#18667,#18668) ;
#15011=AXIS2_PLACEMENT_3D('',#23311,#18670,#18671) ;
#15012=AXIS2_PLACEMENT_3D('',#23312,#18672,#18673) ;
#15013=AXIS2_PLACEMENT_3D('',#23314,#18674,#18675) ;
#15014=AXIS2_PLACEMENT_3D('',#23317,#18677,#18678) ;
#15015=AXIS2_PLACEMENT_3D('',#23318,#18679,#18680) ;
#15016=AXIS2_PLACEMENT_3D('',#23319,#18681,#18682) ;
#15017=AXIS2_PLACEMENT_3D('',#23322,#18683,#18684) ;
#15018=AXIS2_PLACEMENT_3D('',#23328,#18688,#18689) ;
#15019=AXIS2_PLACEMENT_3D('',#23334,#18693,#18694) ;
#15020=AXIS2_PLACEMENT_3D('',#23340,#18698,#18699) ;
#15021=AXIS2_PLACEMENT_3D('',#23341,#18700,#18701) ;
#15022=AXIS2_PLACEMENT_3D('',#23343,#18703,#18704) ;
#15023=AXIS2_PLACEMENT_3D('',#23344,#18705,#18706) ;
#15024=AXIS2_PLACEMENT_3D('',#23347,#18707,#18708) ;
#15025=AXIS2_PLACEMENT_3D('',#23353,#18712,#18713) ;
#15026=AXIS2_PLACEMENT_3D('',#23359,#18717,#18718) ;
#15027=AXIS2_PLACEMENT_3D('',#23365,#18722,#18723) ;
#15028=AXIS2_PLACEMENT_3D('',#23366,#18724,#18725) ;
#15029=AXIS2_PLACEMENT_3D('',#23368,#18727,#18728) ;
#15030=AXIS2_PLACEMENT_3D('',#23369,#18729,#18730) ;
#15031=AXIS2_PLACEMENT_3D('',#23372,#18731,#18732) ;
#15032=AXIS2_PLACEMENT_3D('',#23378,#18736,#18737) ;
#15033=AXIS2_PLACEMENT_3D('',#23384,#18741,#18742) ;
#15034=AXIS2_PLACEMENT_3D('',#23390,#18746,#18747) ;
#15035=AXIS2_PLACEMENT_3D('',#23391,#18748,#18749) ;
#15036=AXIS2_PLACEMENT_3D('',#23393,#18751,#18752) ;
#15037=AXIS2_PLACEMENT_3D('',#23394,#18753,#18754) ;
#15038=AXIS2_PLACEMENT_3D('',#23397,#18755,#18756) ;
#15039=AXIS2_PLACEMENT_3D('',#23403,#18760,#18761) ;
#15040=AXIS2_PLACEMENT_3D('',#23409,#18765,#18766) ;
#15041=AXIS2_PLACEMENT_3D('',#23415,#18770,#18771) ;
#15042=AXIS2_PLACEMENT_3D('',#23416,#18772,#18773) ;
#15043=AXIS2_PLACEMENT_3D('',#23418,#18775,#18776) ;
#15044=AXIS2_PLACEMENT_3D('',#23419,#18777,#18778) ;
#15045=AXIS2_PLACEMENT_3D('',#23422,#18779,#18780) ;
#15046=AXIS2_PLACEMENT_3D('',#23429,#18784,#18785) ;
#15047=AXIS2_PLACEMENT_3D('',#23430,#18786,#18787) ;
#15048=AXIS2_PLACEMENT_3D('',#23436,#18791,#18792) ;
#15049=AXIS2_PLACEMENT_3D('',#23442,#18796,#18797) ;
#15050=AXIS2_PLACEMENT_3D('',#23444,#18798,#18799) ;
#15051=AXIS2_PLACEMENT_3D('',#23446,#18801,#18802) ;
#15052=AXIS2_PLACEMENT_3D('',#23447,#18803,#18804) ;
#15053=AXIS2_PLACEMENT_3D('',#23448,#18805,#18806) ;
#15054=AXIS2_PLACEMENT_3D('',#23451,#18807,#18808) ;
#15055=AXIS2_PLACEMENT_3D('',#23457,#18812,#18813) ;
#15056=AXIS2_PLACEMENT_3D('',#23463,#18817,#18818) ;
#15057=AXIS2_PLACEMENT_3D('',#23469,#18822,#18823) ;
#15058=AXIS2_PLACEMENT_3D('',#23470,#18824,#18825) ;
#15059=AXIS2_PLACEMENT_3D('',#23472,#18827,#18828) ;
#15060=AXIS2_PLACEMENT_3D('',#23473,#18829,#18830) ;
#15061=AXIS2_PLACEMENT_3D('',#23476,#18831,#18832) ;
#15062=AXIS2_PLACEMENT_3D('',#23482,#18836,#18837) ;
#15063=AXIS2_PLACEMENT_3D('',#23488,#18841,#18842) ;
#15064=AXIS2_PLACEMENT_3D('',#23494,#18846,#18847) ;
#15065=AXIS2_PLACEMENT_3D('',#23495,#18848,#18849) ;
#15066=AXIS2_PLACEMENT_3D('',#23497,#18851,#18852) ;
#15067=AXIS2_PLACEMENT_3D('',#23498,#18853,#18854) ;
#15068=AXIS2_PLACEMENT_3D('',#23501,#18855,#18856) ;
#15069=AXIS2_PLACEMENT_3D('',#23507,#18860,#18861) ;
#15070=AXIS2_PLACEMENT_3D('',#23513,#18865,#18866) ;
#15071=AXIS2_PLACEMENT_3D('',#23519,#18870,#18871) ;
#15072=AXIS2_PLACEMENT_3D('',#23520,#18872,#18873) ;
#15073=AXIS2_PLACEMENT_3D('',#23522,#18875,#18876) ;
#15074=AXIS2_PLACEMENT_3D('',#23523,#18877,#18878) ;
#15075=AXIS2_PLACEMENT_3D('',#23526,#18879,#18880) ;
#15076=AXIS2_PLACEMENT_3D('',#23532,#18884,#18885) ;
#15077=AXIS2_PLACEMENT_3D('',#23538,#18889,#18890) ;
#15078=AXIS2_PLACEMENT_3D('',#23544,#18894,#18895) ;
#15079=AXIS2_PLACEMENT_3D('',#23545,#18896,#18897) ;
#15080=AXIS2_PLACEMENT_3D('',#23547,#18899,#18900) ;
#15081=AXIS2_PLACEMENT_3D('',#23548,#18901,#18902) ;
#15082=AXIS2_PLACEMENT_3D('',#23551,#18903,#18904) ;
#15083=AXIS2_PLACEMENT_3D('',#23557,#18908,#18909) ;
#15084=AXIS2_PLACEMENT_3D('',#23563,#18913,#18914) ;
#15085=AXIS2_PLACEMENT_3D('',#23569,#18918,#18919) ;
#15086=AXIS2_PLACEMENT_3D('',#23570,#18920,#18921) ;
#15087=AXIS2_PLACEMENT_3D('',#23572,#18923,#18924) ;
#15088=AXIS2_PLACEMENT_3D('',#23573,#18925,#18926) ;
#15089=AXIS2_PLACEMENT_3D('',#23575,#18927,#18928) ;
#15090=AXIS2_PLACEMENT_3D('',#23579,#18931,#18932) ;
#15091=AXIS2_PLACEMENT_3D('',#23580,#18933,#18934) ;
#15092=AXIS2_PLACEMENT_3D('',#23581,#18935,#18936) ;
#18663=DIRECTION('axis',(0.,0.,1.)) ;
#18664=DIRECTION('refdir',(1.,0.,0.)) ;
#18665=DIRECTION('center_axis',(0.,1.,0.)) ;
#18666=DIRECTION('ref_axis',(1.,0.,0.)) ;
#18667=DIRECTION('center_axis',(0.,1.,0.)) ;
#18668=DIRECTION('ref_axis',(1.,0.,0.)) ;
#18669=DIRECTION('',(0.,1.,0.)) ;
#18670=DIRECTION('center_axis',(0.,-1.,0.)) ;
#18671=DIRECTION('ref_axis',(1.,0.,0.)) ;
#18672=DIRECTION('center_axis',(0.,1.,0.)) ;
#18673=DIRECTION('ref_axis',(1.,0.,0.)) ;
#18674=DIRECTION('center_axis',(0.,1.,0.)) ;
#18675=DIRECTION('ref_axis',(1.,0.,0.)) ;
#18676=DIRECTION('',(0.,-1.,0.)) ;
#18677=DIRECTION('center_axis',(0.,-1.,0.)) ;
#18678=DIRECTION('ref_axis',(1.,0.,0.)) ;
#18679=DIRECTION('center_axis',(0.,-1.,0.)) ;
#18680=DIRECTION('ref_axis',(-1.,0.,0.)) ;
#18681=DIRECTION('center_axis',(0.,1.,0.)) ;
#18682=DIRECTION('ref_axis',(0.587785252292473,0.,0.809016994374947)) ;
#18683=DIRECTION('center_axis',(0.,-1.,0.)) ;
#18684=DIRECTION('ref_axis',(1.,0.,0.)) ;
#18685=DIRECTION('',(-0.809016994374947,0.,0.587785252292473)) ;
#18686=DIRECTION('',(-0.587785252292473,0.,-0.809016994374947)) ;
#18687=DIRECTION('',(0.809016994374947,0.,-0.587785252292473)) ;
#18688=DIRECTION('center_axis',(0.587785252292473,0.,0.809016994374947)) ;
#18689=DIRECTION('ref_axis',(0.809016994374947,0.,-0.587785252292473)) ;
#18690=DIRECTION('',(0.,-1.,0.)) ;
#18691=DIRECTION('',(0.809016994374947,0.,-0.587785252292473)) ;
#18692=DIRECTION('',(0.,-1.,0.)) ;
#18693=DIRECTION('center_axis',(0.587785252292473,0.,0.809016994374947)) ;
#18694=DIRECTION('ref_axis',(0.809016994374947,0.,-0.587785252292473)) ;
#18695=DIRECTION('',(0.,1.,0.)) ;
#18696=DIRECTION('',(0.,1.,0.)) ;
#18697=DIRECTION('',(-0.809016994374947,0.,0.587785252292473)) ;
#18698=DIRECTION('center_axis',(0.,-1.,0.)) ;
#18699=DIRECTION('ref_axis',(-0.587785252292473,0.,-0.809016994374947)) ;
#18700=DIRECTION('center_axis',(0.,1.,0.)) ;
#18701=DIRECTION('ref_axis',(1.,0.,0.)) ;
#18702=DIRECTION('',(-0.587785252292473,0.,-0.809016994374947)) ;
#18703=DIRECTION('center_axis',(-0.809016994374947,0.,0.587785252292473)) ;
#18704=DIRECTION('ref_axis',(0.587785252292473,0.,0.809016994374947)) ;
#18705=DIRECTION('center_axis',(0.,1.,0.)) ;
#18706=DIRECTION('ref_axis',(0.951056516295154,0.,0.309016994374947)) ;
#18707=DIRECTION('center_axis',(0.,-1.,0.)) ;
#18708=DIRECTION('ref_axis',(1.,0.,0.)) ;
#18709=DIRECTION('',(-0.309016994374947,0.,0.951056516295154)) ;
#18710=DIRECTION('',(-0.951056516295154,0.,-0.309016994374947)) ;
#18711=DIRECTION('',(0.309016994374947,0.,-0.951056516295154)) ;
#18712=DIRECTION('center_axis',(0.951056516295154,0.,0.309016994374947)) ;
#18713=DIRECTION('ref_axis',(0.309016994374947,0.,-0.951056516295154)) ;
#18714=DIRECTION('',(0.,-1.,0.)) ;
#18715=DIRECTION('',(0.309016994374947,0.,-0.951056516295154)) ;
#18716=DIRECTION('',(0.,-1.,0.)) ;
#18717=DIRECTION('center_axis',(0.951056516295154,0.,0.309016994374947)) ;
#18718=DIRECTION('ref_axis',(0.309016994374947,0.,-0.951056516295154)) ;
#18719=DIRECTION('',(0.,1.,0.)) ;
#18720=DIRECTION('',(0.,1.,0.)) ;
#18721=DIRECTION('',(-0.309016994374947,0.,0.951056516295154)) ;
#18722=DIRECTION('center_axis',(0.,-1.,0.)) ;
#18723=DIRECTION('ref_axis',(-0.951056516295154,0.,-0.309016994374947)) ;
#18724=DIRECTION('center_axis',(0.,1.,0.)) ;
#18725=DIRECTION('ref_axis',(1.,0.,0.)) ;
#18726=DIRECTION('',(-0.951056516295154,0.,-0.309016994374947)) ;
#18727=DIRECTION('center_axis',(-0.309016994374947,0.,0.951056516295154)) ;
#18728=DIRECTION('ref_axis',(0.951056516295154,0.,0.309016994374947)) ;
#18729=DIRECTION('center_axis',(0.,1.,0.)) ;
#18730=DIRECTION('ref_axis',(0.951056516295154,0.,-0.309016994374948)) ;
#18731=DIRECTION('center_axis',(0.,-1.,0.)) ;
#18732=DIRECTION('ref_axis',(1.,0.,0.)) ;
#18733=DIRECTION('',(0.309016994374948,0.,0.951056516295154)) ;
#18734=DIRECTION('',(-0.951056516295154,0.,0.309016994374948)) ;
#18735=DIRECTION('',(-0.309016994374948,0.,-0.951056516295154)) ;
#18736=DIRECTION('center_axis',(0.951056516295154,0.,-0.309016994374948)) ;
#18737=DIRECTION('ref_axis',(-0.309016994374948,0.,-0.951056516295154)) ;
#18738=DIRECTION('',(0.,-1.,0.)) ;
#18739=DIRECTION('',(-0.309016994374948,0.,-0.951056516295154)) ;
#18740=DIRECTION('',(0.,-1.,0.)) ;
#18741=DIRECTION('center_axis',(0.951056516295154,0.,-0.309016994374948)) ;
#18742=DIRECTION('ref_axis',(-0.309016994374948,0.,-0.951056516295154)) ;
#18743=DIRECTION('',(0.,1.,0.)) ;
#18744=DIRECTION('',(0.,1.,0.)) ;
#18745=DIRECTION('',(0.309016994374948,0.,0.951056516295154)) ;
#18746=DIRECTION('center_axis',(0.,-1.,0.)) ;
#18747=DIRECTION('ref_axis',(-0.951056516295154,0.,0.309016994374948)) ;
#18748=DIRECTION('center_axis',(0.,1.,0.)) ;
#18749=DIRECTION('ref_axis',(1.,0.,0.)) ;
#18750=DIRECTION('',(-0.951056516295154,0.,0.309016994374948)) ;
#18751=DIRECTION('center_axis',(0.309016994374948,0.,0.951056516295154)) ;
#18752=DIRECTION('ref_axis',(0.951056516295154,0.,-0.309016994374948)) ;
#18753=DIRECTION('center_axis',(0.,1.,0.)) ;
#18754=DIRECTION('ref_axis',(0.587785252292473,0.,-0.809016994374948)) ;
#18755=DIRECTION('center_axis',(0.,-1.,0.)) ;
#18756=DIRECTION('ref_axis',(1.,0.,0.)) ;
#18757=DIRECTION('',(0.809016994374948,0.,0.587785252292473)) ;
#18758=DIRECTION('',(-0.587785252292473,0.,0.809016994374948)) ;
#18759=DIRECTION('',(-0.809016994374948,0.,-0.587785252292473)) ;
#18760=DIRECTION('center_axis',(0.587785252292473,0.,-0.809016994374948)) ;
#18761=DIRECTION('ref_axis',(-0.809016994374948,0.,-0.587785252292473)) ;
#18762=DIRECTION('',(0.,-1.,0.)) ;
#18763=DIRECTION('',(-0.809016994374948,0.,-0.587785252292473)) ;
#18764=DIRECTION('',(0.,-1.,0.)) ;
#18765=DIRECTION('center_axis',(0.587785252292473,0.,-0.809016994374948)) ;
#18766=DIRECTION('ref_axis',(-0.809016994374948,0.,-0.587785252292473)) ;
#18767=DIRECTION('',(0.,1.,0.)) ;
#18768=DIRECTION('',(0.,1.,0.)) ;
#18769=DIRECTION('',(0.809016994374948,0.,0.587785252292473)) ;
#18770=DIRECTION('center_axis',(0.,-1.,0.)) ;
#18771=DIRECTION('ref_axis',(-0.587785252292473,0.,0.809016994374948)) ;
#18772=DIRECTION('center_axis',(0.,1.,0.)) ;
#18773=DIRECTION('ref_axis',(1.,0.,0.)) ;
#18774=DIRECTION('',(-0.587785252292473,0.,0.809016994374948)) ;
#18775=DIRECTION('center_axis',(0.809016994374948,0.,0.587785252292473)) ;
#18776=DIRECTION('ref_axis',(0.587785252292473,0.,-0.809016994374948)) ;
#18777=DIRECTION('center_axis',(0.,1.,0.)) ;
#18778=DIRECTION('ref_axis',(-1.22464679914735E-16,0.,-1.)) ;
#18779=DIRECTION('center_axis',(0.,-1.,0.)) ;
#18780=DIRECTION('ref_axis',(1.,0.,0.)) ;
#18781=DIRECTION('',(1.,0.,-1.22464679914735E-16)) ;
#18782=DIRECTION('',(1.22464679914735E-16,0.,1.)) ;
#18783=DIRECTION('',(-1.,0.,1.22464679914735E-16)) ;
#18784=DIRECTION('center_axis',(0.,-1.,0.)) ;
#18785=DIRECTION('ref_axis',(1.,0.,0.)) ;
#18786=DIRECTION('center_axis',(-1.22464679914735E-16,0.,-1.)) ;
#18787=DIRECTION('ref_axis',(-1.,0.,1.22464679914735E-16)) ;
#18788=DIRECTION('',(0.,-1.,0.)) ;
#18789=DIRECTION('',(-1.,0.,1.22464679914735E-16)) ;
#18790=DIRECTION('',(0.,-1.,0.)) ;
#18791=DIRECTION('center_axis',(-1.22464679914735E-16,0.,-1.)) ;
#18792=DIRECTION('ref_axis',(-1.,0.,1.22464679914735E-16)) ;
#18793=DIRECTION('',(0.,1.,0.)) ;
#18794=DIRECTION('',(0.,1.,0.)) ;
#18795=DIRECTION('',(1.,0.,-1.22464679914735E-16)) ;
#18796=DIRECTION('center_axis',(0.,-1.,0.)) ;
#18797=DIRECTION('ref_axis',(1.22464679914735E-16,0.,1.)) ;
#18798=DIRECTION('center_axis',(0.,1.,0.)) ;
#18799=DIRECTION('ref_axis',(1.,0.,0.)) ;
#18800=DIRECTION('',(1.22464679914735E-16,0.,1.)) ;
#18801=DIRECTION('center_axis',(0.,1.,0.)) ;
#18802=DIRECTION('ref_axis',(1.,0.,0.)) ;
#18803=DIRECTION('center_axis',(1.,0.,-1.22464679914735E-16)) ;
#18804=DIRECTION('ref_axis',(-1.22464679914735E-16,0.,-1.)) ;
#18805=DIRECTION('center_axis',(0.,1.,0.)) ;
#18806=DIRECTION('ref_axis',(-0.587785252292473,0.,-0.809016994374947)) ;
#18807=DIRECTION('center_axis',(0.,-1.,0.)) ;
#18808=DIRECTION('ref_axis',(1.,0.,0.)) ;
#18809=DIRECTION('',(0.809016994374947,0.,-0.587785252292473)) ;
#18810=DIRECTION('',(0.587785252292473,0.,0.809016994374947)) ;
#18811=DIRECTION('',(-0.809016994374947,0.,0.587785252292473)) ;
#18812=DIRECTION('center_axis',(-0.587785252292473,0.,-0.809016994374947)) ;
#18813=DIRECTION('ref_axis',(-0.809016994374947,0.,0.587785252292473)) ;
#18814=DIRECTION('',(0.,-1.,0.)) ;
#18815=DIRECTION('',(-0.809016994374947,0.,0.587785252292473)) ;
#18816=DIRECTION('',(0.,-1.,0.)) ;
#18817=DIRECTION('center_axis',(-0.587785252292473,0.,-0.809016994374947)) ;
#18818=DIRECTION('ref_axis',(-0.809016994374947,0.,0.587785252292473)) ;
#18819=DIRECTION('',(0.,1.,0.)) ;
#18820=DIRECTION('',(0.,1.,0.)) ;
#18821=DIRECTION('',(0.809016994374947,0.,-0.587785252292473)) ;
#18822=DIRECTION('center_axis',(0.,-1.,0.)) ;
#18823=DIRECTION('ref_axis',(0.587785252292473,0.,0.809016994374947)) ;
#18824=DIRECTION('center_axis',(0.,1.,0.)) ;
#18825=DIRECTION('ref_axis',(1.,0.,0.)) ;
#18826=DIRECTION('',(0.587785252292473,0.,0.809016994374947)) ;
#18827=DIRECTION('center_axis',(0.809016994374947,0.,-0.587785252292473)) ;
#18828=DIRECTION('ref_axis',(-0.587785252292473,0.,-0.809016994374947)) ;
#18829=DIRECTION('center_axis',(0.,1.,0.)) ;
#18830=DIRECTION('ref_axis',(-0.951056516295154,0.,-0.309016994374947)) ;
#18831=DIRECTION('center_axis',(0.,-1.,0.)) ;
#18832=DIRECTION('ref_axis',(1.,0.,0.)) ;
#18833=DIRECTION('',(0.309016994374947,0.,-0.951056516295154)) ;
#18834=DIRECTION('',(0.951056516295154,0.,0.309016994374947)) ;
#18835=DIRECTION('',(-0.309016994374947,0.,0.951056516295154)) ;
#18836=DIRECTION('center_axis',(-0.951056516295154,0.,-0.309016994374947)) ;
#18837=DIRECTION('ref_axis',(-0.309016994374947,0.,0.951056516295154)) ;
#18838=DIRECTION('',(0.,-1.,0.)) ;
#18839=DIRECTION('',(-0.309016994374947,0.,0.951056516295154)) ;
#18840=DIRECTION('',(0.,-1.,0.)) ;
#18841=DIRECTION('center_axis',(-0.951056516295154,0.,-0.309016994374947)) ;
#18842=DIRECTION('ref_axis',(-0.309016994374947,0.,0.951056516295154)) ;
#18843=DIRECTION('',(0.,1.,0.)) ;
#18844=DIRECTION('',(0.,1.,0.)) ;
#18845=DIRECTION('',(0.309016994374947,0.,-0.951056516295154)) ;
#18846=DIRECTION('center_axis',(0.,-1.,0.)) ;
#18847=DIRECTION('ref_axis',(0.951056516295154,0.,0.309016994374947)) ;
#18848=DIRECTION('center_axis',(0.,1.,0.)) ;
#18849=DIRECTION('ref_axis',(1.,0.,0.)) ;
#18850=DIRECTION('',(0.951056516295154,0.,0.309016994374947)) ;
#18851=DIRECTION('center_axis',(0.309016994374947,0.,-0.951056516295154)) ;
#18852=DIRECTION('ref_axis',(-0.951056516295154,0.,-0.309016994374947)) ;
#18853=DIRECTION('center_axis',(0.,1.,0.)) ;
#18854=DIRECTION('ref_axis',(-0.951056516295154,0.,0.309016994374948)) ;
#18855=DIRECTION('center_axis',(0.,-1.,0.)) ;
#18856=DIRECTION('ref_axis',(1.,0.,0.)) ;
#18857=DIRECTION('',(-0.309016994374948,0.,-0.951056516295154)) ;
#18858=DIRECTION('',(0.951056516295154,0.,-0.309016994374948)) ;
#18859=DIRECTION('',(0.309016994374948,0.,0.951056516295154)) ;
#18860=DIRECTION('center_axis',(-0.951056516295154,0.,0.309016994374948)) ;
#18861=DIRECTION('ref_axis',(0.309016994374948,0.,0.951056516295154)) ;
#18862=DIRECTION('',(0.,-1.,0.)) ;
#18863=DIRECTION('',(0.309016994374948,0.,0.951056516295154)) ;
#18864=DIRECTION('',(0.,-1.,0.)) ;
#18865=DIRECTION('center_axis',(-0.951056516295154,0.,0.309016994374948)) ;
#18866=DIRECTION('ref_axis',(0.309016994374948,0.,0.951056516295154)) ;
#18867=DIRECTION('',(0.,1.,0.)) ;
#18868=DIRECTION('',(0.,1.,0.)) ;
#18869=DIRECTION('',(-0.309016994374948,0.,-0.951056516295154)) ;
#18870=DIRECTION('center_axis',(0.,-1.,0.)) ;
#18871=DIRECTION('ref_axis',(0.951056516295154,0.,-0.309016994374948)) ;
#18872=DIRECTION('center_axis',(0.,1.,0.)) ;
#18873=DIRECTION('ref_axis',(1.,0.,0.)) ;
#18874=DIRECTION('',(0.951056516295154,0.,-0.309016994374948)) ;
#18875=DIRECTION('center_axis',(-0.309016994374948,0.,-0.951056516295154)) ;
#18876=DIRECTION('ref_axis',(-0.951056516295154,0.,0.309016994374948)) ;
#18877=DIRECTION('center_axis',(0.,1.,0.)) ;
#18878=DIRECTION('ref_axis',(-0.587785252292473,0.,0.809016994374947)) ;
#18879=DIRECTION('center_axis',(0.,-1.,0.)) ;
#18880=DIRECTION('ref_axis',(1.,0.,0.)) ;
#18881=DIRECTION('',(-0.809016994374947,0.,-0.587785252292473)) ;
#18882=DIRECTION('',(0.587785252292473,0.,-0.809016994374947)) ;
#18883=DIRECTION('',(0.809016994374947,0.,0.587785252292473)) ;
#18884=DIRECTION('center_axis',(-0.587785252292473,0.,0.809016994374947)) ;
#18885=DIRECTION('ref_axis',(0.809016994374947,0.,0.587785252292473)) ;
#18886=DIRECTION('',(0.,-1.,0.)) ;
#18887=DIRECTION('',(0.809016994374947,0.,0.587785252292473)) ;
#18888=DIRECTION('',(0.,-1.,0.)) ;
#18889=DIRECTION('center_axis',(-0.587785252292473,0.,0.809016994374947)) ;
#18890=DIRECTION('ref_axis',(0.809016994374947,0.,0.587785252292473)) ;
#18891=DIRECTION('',(0.,1.,0.)) ;
#18892=DIRECTION('',(0.,1.,0.)) ;
#18893=DIRECTION('',(-0.809016994374947,0.,-0.587785252292473)) ;
#18894=DIRECTION('center_axis',(0.,-1.,0.)) ;
#18895=DIRECTION('ref_axis',(0.587785252292473,0.,-0.809016994374947)) ;
#18896=DIRECTION('center_axis',(0.,1.,0.)) ;
#18897=DIRECTION('ref_axis',(1.,0.,0.)) ;
#18898=DIRECTION('',(0.587785252292473,0.,-0.809016994374947)) ;
#18899=DIRECTION('center_axis',(-0.809016994374947,0.,-0.587785252292473)) ;
#18900=DIRECTION('ref_axis',(-0.587785252292473,0.,0.809016994374947)) ;
#18901=DIRECTION('center_axis',(0.,1.,0.)) ;
#18902=DIRECTION('ref_axis',(0.,0.,1.)) ;
#18903=DIRECTION('center_axis',(0.,-1.,0.)) ;
#18904=DIRECTION('ref_axis',(1.,0.,0.)) ;
#18905=DIRECTION('',(-1.,0.,0.)) ;
#18906=DIRECTION('',(0.,0.,-1.)) ;
#18907=DIRECTION('',(1.,0.,0.)) ;
#18908=DIRECTION('center_axis',(0.,0.,1.)) ;
#18909=DIRECTION('ref_axis',(1.,0.,0.)) ;
#18910=DIRECTION('',(0.,-1.,0.)) ;
#18911=DIRECTION('',(1.,0.,0.)) ;
#18912=DIRECTION('',(0.,-1.,0.)) ;
#18913=DIRECTION('center_axis',(0.,0.,1.)) ;
#18914=DIRECTION('ref_axis',(1.,0.,0.)) ;
#18915=DIRECTION('',(0.,1.,0.)) ;
#18916=DIRECTION('',(0.,1.,0.)) ;
#18917=DIRECTION('',(-1.,0.,0.)) ;
#18918=DIRECTION('center_axis',(0.,-1.,0.)) ;
#18919=DIRECTION('ref_axis',(0.,0.,-1.)) ;
#18920=DIRECTION('center_axis',(0.,1.,0.)) ;
#18921=DIRECTION('ref_axis',(1.,0.,0.)) ;
#18922=DIRECTION('',(0.,0.,-1.)) ;
#18923=DIRECTION('center_axis',(-1.,0.,0.)) ;
#18924=DIRECTION('ref_axis',(0.,0.,1.)) ;
#18925=DIRECTION('center_axis',(0.,1.,0.)) ;
#18926=DIRECTION('ref_axis',(1.,0.,0.)) ;
#18927=DIRECTION('center_axis',(0.,1.,0.)) ;
#18928=DIRECTION('ref_axis',(1.,0.,0.)) ;
#18929=DIRECTION('',(0.,-1.,0.)) ;
#18930=DIRECTION('',(0.,-1.,0.)) ;
#18931=DIRECTION('center_axis',(0.,-1.,0.)) ;
#18932=DIRECTION('ref_axis',(1.,0.,0.)) ;
#18933=DIRECTION('center_axis',(0.,-1.,0.)) ;
#18934=DIRECTION('ref_axis',(-1.,0.,0.)) ;
#18935=DIRECTION('center_axis',(0.,1.,0.)) ;
#18936=DIRECTION('ref_axis',(1.,0.,0.)) ;
#23305=CARTESIAN_POINT('',(0.,0.,0.)) ;
#23306=CARTESIAN_POINT('Origin',(-23.,2.1,-2.2)) ;
#23307=CARTESIAN_POINT('',(-23.4,1.6,-2.2)) ;
#23308=CARTESIAN_POINT('Origin',(-23.,1.6,-2.2)) ;
#23309=CARTESIAN_POINT('',(-23.4,2.6,-2.2)) ;
#23310=CARTESIAN_POINT('',(-23.4,2.1,-2.2)) ;
#23311=CARTESIAN_POINT('Origin',(-23.,2.6,-2.2)) ;
#23312=CARTESIAN_POINT('Origin',(-23.,2.1,-2.2)) ;
#23313=CARTESIAN_POINT('',(-23.8,2.,-2.2)) ;
#23314=CARTESIAN_POINT('Origin',(-23.,2.,-2.2)) ;
#23315=CARTESIAN_POINT('',(-23.8,1.6,-2.2)) ;
#23316=CARTESIAN_POINT('',(-23.8,2.1,-2.2)) ;
#23317=CARTESIAN_POINT('Origin',(-23.,1.6,-2.2)) ;
#23318=CARTESIAN_POINT('Origin',(-23.,1.6,-2.2)) ;
#23319=CARTESIAN_POINT('Origin',(-21.6651219592813,2.05,-3.16984566628258)) ;
#23320=CARTESIAN_POINT('',(-21.9148668248458,2.05,-3.23560899579898)) ;
#23321=CARTESIAN_POINT('',(-21.6797527239288,2.05,-2.912002198049)) ;
#23322=CARTESIAN_POINT('Origin',(-23.,2.05,-2.2)) ;
#23323=CARTESIAN_POINT('',(-21.6208756108648,2.05,-3.44920611561607)) ;
#23324=CARTESIAN_POINT('',(-21.7826790097398,2.05,-3.33164906515757)) ;
#23325=CARTESIAN_POINT('',(-21.3857615099479,2.05,-3.12559931786609)) ;
#23326=CARTESIAN_POINT('',(-21.5033185604063,2.05,-3.28740271674108)) ;
#23327=CARTESIAN_POINT('',(-21.5475649088228,2.05,-3.00804226740759)) ;
#23328=CARTESIAN_POINT('Origin',(-21.7826790097398,2.3,-3.33164906515757)) ;
#23329=CARTESIAN_POINT('',(-21.9148668248458,2.55,-3.23560899579898)) ;
#23330=CARTESIAN_POINT('',(-21.9148668248458,2.3,-3.23560899579898)) ;
#23331=CARTESIAN_POINT('',(-21.6208756108648,2.55,-3.44920611561607)) ;
#23332=CARTESIAN_POINT('',(-21.7826790097398,2.55,-3.33164906515757)) ;
#23333=CARTESIAN_POINT('',(-21.6208756108648,2.3,-3.44920611561607)) ;
#23334=CARTESIAN_POINT('Origin',(-21.5475649088228,2.3,-3.00804226740759)) ;
#23335=CARTESIAN_POINT('',(-21.6797527239288,2.55,-2.912002198049)) ;
#23336=CARTESIAN_POINT('',(-21.6797527239288,2.3,-2.912002198049)) ;
#23337=CARTESIAN_POINT('',(-21.3857615099479,2.55,-3.12559931786609)) ;
#23338=CARTESIAN_POINT('',(-21.3857615099479,2.3,-3.12559931786609)) ;
#23339=CARTESIAN_POINT('',(-21.5475649088228,2.55,-3.00804226740759)) ;
#23340=CARTESIAN_POINT('Origin',(-21.6651219592813,2.55,-3.16984566628258)) ;
#23341=CARTESIAN_POINT('Origin',(-23.,2.55,-2.2)) ;
#23342=CARTESIAN_POINT('',(-21.5033185604063,2.55,-3.28740271674108)) ;
#23343=CARTESIAN_POINT('Origin',(-21.5033185604063,2.3,-3.28740271674108)) ;
#23344=CARTESIAN_POINT('Origin',(-22.4901219592813,2.05,-3.769243251887)) ;
#23345=CARTESIAN_POINT('',(-22.7308245150123,2.05,-3.67565055425789)) ;
#23346=CARTESIAN_POINT('',(-22.3504019084942,2.05,-3.55204375650791)) ;
#23347=CARTESIAN_POINT('Origin',(-23.,2.05,-2.2)) ;
#23348=CARTESIAN_POINT('',(-22.6185298636654,2.05,-4.02125795402102)) ;
#23349=CARTESIAN_POINT('',(-22.6803332625404,2.05,-3.83104665076199)) ;
#23350=CARTESIAN_POINT('',(-22.2381072571473,2.05,-3.89765115627104)) ;
#23351=CARTESIAN_POINT('',(-22.4283185604063,2.05,-3.95945455514603)) ;
#23352=CARTESIAN_POINT('',(-22.2999106560223,2.05,-3.70743985301201)) ;
#23353=CARTESIAN_POINT('Origin',(-22.6803332625404,2.3,-3.83104665076199)) ;
#23354=CARTESIAN_POINT('',(-22.7308245150123,2.55,-3.67565055425789)) ;
#23355=CARTESIAN_POINT('',(-22.7308245150123,2.3,-3.67565055425789)) ;
#23356=CARTESIAN_POINT('',(-22.6185298636654,2.55,-4.02125795402102)) ;
#23357=CARTESIAN_POINT('',(-22.6803332625404,2.55,-3.83104665076199)) ;
#23358=CARTESIAN_POINT('',(-22.6185298636654,2.3,-4.02125795402102)) ;
#23359=CARTESIAN_POINT('Origin',(-22.2999106560223,2.3,-3.70743985301201)) ;
#23360=CARTESIAN_POINT('',(-22.3504019084942,2.55,-3.55204375650791)) ;
#23361=CARTESIAN_POINT('',(-22.3504019084942,2.3,-3.55204375650791)) ;
#23362=CARTESIAN_POINT('',(-22.2381072571473,2.55,-3.89765115627104)) ;
#23363=CARTESIAN_POINT('',(-22.2381072571473,2.3,-3.89765115627104)) ;
#23364=CARTESIAN_POINT('',(-22.2999106560223,2.55,-3.70743985301201)) ;
#23365=CARTESIAN_POINT('Origin',(-22.4901219592813,2.55,-3.769243251887)) ;
#23366=CARTESIAN_POINT('Origin',(-23.,2.55,-2.2)) ;
#23367=CARTESIAN_POINT('',(-22.4283185604063,2.55,-3.95945455514603)) ;
#23368=CARTESIAN_POINT('Origin',(-22.4283185604063,2.3,-3.95945455514603)) ;
#23369=CARTESIAN_POINT('Origin',(-23.5098780407187,2.05,-3.769243251887)) ;
#23370=CARTESIAN_POINT('',(-23.6495980915058,2.05,-3.55204375650791)) ;
#23371=CARTESIAN_POINT('',(-23.2691754849877,2.05,-3.67565055425789)) ;
#23372=CARTESIAN_POINT('Origin',(-23.,2.05,-2.2)) ;
#23373=CARTESIAN_POINT('',(-23.7618927428527,2.05,-3.89765115627104)) ;
#23374=CARTESIAN_POINT('',(-23.7000893439777,2.05,-3.70743985301201)) ;
#23375=CARTESIAN_POINT('',(-23.3814701363346,2.05,-4.02125795402102)) ;
#23376=CARTESIAN_POINT('',(-23.5716814395937,2.05,-3.95945455514603)) ;
#23377=CARTESIAN_POINT('',(-23.3196667374596,2.05,-3.83104665076199)) ;
#23378=CARTESIAN_POINT('Origin',(-23.7000893439777,2.3,-3.70743985301201)) ;
#23379=CARTESIAN_POINT('',(-23.6495980915058,2.55,-3.55204375650791)) ;
#23380=CARTESIAN_POINT('',(-23.6495980915058,2.3,-3.55204375650791)) ;
#23381=CARTESIAN_POINT('',(-23.7618927428527,2.55,-3.89765115627104)) ;
#23382=CARTESIAN_POINT('',(-23.7000893439777,2.55,-3.70743985301201)) ;
#23383=CARTESIAN_POINT('',(-23.7618927428527,2.3,-3.89765115627104)) ;
#23384=CARTESIAN_POINT('Origin',(-23.3196667374596,2.3,-3.83104665076199)) ;
#23385=CARTESIAN_POINT('',(-23.2691754849877,2.55,-3.67565055425789)) ;
#23386=CARTESIAN_POINT('',(-23.2691754849877,2.3,-3.67565055425789)) ;
#23387=CARTESIAN_POINT('',(-23.3814701363346,2.55,-4.02125795402102)) ;
#23388=CARTESIAN_POINT('',(-23.3814701363346,2.3,-4.02125795402102)) ;
#23389=CARTESIAN_POINT('',(-23.3196667374596,2.55,-3.83104665076199)) ;
#23390=CARTESIAN_POINT('Origin',(-23.5098780407187,2.55,-3.769243251887)) ;
#23391=CARTESIAN_POINT('Origin',(-23.,2.55,-2.2)) ;
#23392=CARTESIAN_POINT('',(-23.5716814395937,2.55,-3.95945455514603)) ;
#23393=CARTESIAN_POINT('Origin',(-23.5716814395937,2.3,-3.95945455514603)) ;
#23394=CARTESIAN_POINT('Origin',(-24.3348780407187,2.05,-3.16984566628258)) ;
#23395=CARTESIAN_POINT('',(-24.3202472760712,2.05,-2.912002198049)) ;
#23396=CARTESIAN_POINT('',(-24.0851331751542,2.05,-3.23560899579897)) ;
#23397=CARTESIAN_POINT('Origin',(-23.,2.05,-2.2)) ;
#23398=CARTESIAN_POINT('',(-24.6142384900521,2.05,-3.12559931786609)) ;
#23399=CARTESIAN_POINT('',(-24.4524350911772,2.05,-3.00804226740759)) ;
#23400=CARTESIAN_POINT('',(-24.3791243891352,2.05,-3.44920611561606)) ;
#23401=CARTESIAN_POINT('',(-24.4966814395937,2.05,-3.28740271674108)) ;
#23402=CARTESIAN_POINT('',(-24.2173209902602,2.05,-3.33164906515757)) ;
#23403=CARTESIAN_POINT('Origin',(-24.4524350911772,2.3,-3.00804226740759)) ;
#23404=CARTESIAN_POINT('',(-24.3202472760712,2.55,-2.912002198049)) ;
#23405=CARTESIAN_POINT('',(-24.3202472760712,2.3,-2.912002198049)) ;
#23406=CARTESIAN_POINT('',(-24.6142384900521,2.55,-3.12559931786609)) ;
#23407=CARTESIAN_POINT('',(-24.4524350911772,2.55,-3.00804226740759)) ;
#23408=CARTESIAN_POINT('',(-24.6142384900521,2.3,-3.12559931786609)) ;
#23409=CARTESIAN_POINT('Origin',(-24.2173209902602,2.3,-3.33164906515757)) ;
#23410=CARTESIAN_POINT('',(-24.0851331751542,2.55,-3.23560899579897)) ;
#23411=CARTESIAN_POINT('',(-24.0851331751542,2.3,-3.23560899579897)) ;
#23412=CARTESIAN_POINT('',(-24.3791243891352,2.55,-3.44920611561606)) ;
#23413=CARTESIAN_POINT('',(-24.3791243891352,2.3,-3.44920611561606)) ;
#23414=CARTESIAN_POINT('',(-24.2173209902602,2.55,-3.33164906515757)) ;
#23415=CARTESIAN_POINT('Origin',(-24.3348780407187,2.55,-3.16984566628258)) ;
#23416=CARTESIAN_POINT('Origin',(-23.,2.55,-2.2)) ;
#23417=CARTESIAN_POINT('',(-24.4966814395937,2.55,-3.28740271674108)) ;
#23418=CARTESIAN_POINT('Origin',(-24.4966814395937,2.3,-3.28740271674108)) ;
#23419=CARTESIAN_POINT('Origin',(-24.65,2.05,-2.2)) ;
#23420=CARTESIAN_POINT('',(-24.4866068747319,2.05,-2.)) ;
#23421=CARTESIAN_POINT('',(-24.5,2.05,-2.2)) ;
#23422=CARTESIAN_POINT('Origin',(-23.,2.05,-2.2)) ;
#23423=CARTESIAN_POINT('',(-24.85,2.05,-2.)) ;
#23424=CARTESIAN_POINT('',(-24.65,2.05,-2.)) ;
#23425=CARTESIAN_POINT('',(-24.85,2.05,-2.4)) ;
#23426=CARTESIAN_POINT('',(-24.85,2.05,-2.2)) ;
#23427=CARTESIAN_POINT('',(-24.4866068747319,2.05,-2.4)) ;
#23428=CARTESIAN_POINT('',(-24.65,2.05,-2.4)) ;
#23429=CARTESIAN_POINT('Origin',(-23.,2.05,-2.2)) ;
#23430=CARTESIAN_POINT('Origin',(-24.65,2.3,-2.)) ;
#23431=CARTESIAN_POINT('',(-24.4866068747319,2.55,-2.)) ;
#23432=CARTESIAN_POINT('',(-24.4866068747319,2.3,-2.)) ;
#23433=CARTESIAN_POINT('',(-24.85,2.55,-2.)) ;
#23434=CARTESIAN_POINT('',(-24.65,2.55,-2.)) ;
#23435=CARTESIAN_POINT('',(-24.85,2.3,-2.)) ;
#23436=CARTESIAN_POINT('Origin',(-24.65,2.3,-2.4)) ;
#23437=CARTESIAN_POINT('',(-24.4866068747319,2.55,-2.4)) ;
#23438=CARTESIAN_POINT('',(-24.4866068747319,2.3,-2.4)) ;
#23439=CARTESIAN_POINT('',(-24.85,2.55,-2.4)) ;
#23440=CARTESIAN_POINT('',(-24.85,2.3,-2.4)) ;
#23441=CARTESIAN_POINT('',(-24.65,2.55,-2.4)) ;
#23442=CARTESIAN_POINT('Origin',(-24.65,2.55,-2.2)) ;
#23443=CARTESIAN_POINT('',(-24.5,2.55,-2.2)) ;
#23444=CARTESIAN_POINT('Origin',(-23.,2.55,-2.2)) ;
#23445=CARTESIAN_POINT('',(-24.85,2.55,-2.2)) ;
#23446=CARTESIAN_POINT('Origin',(-23.,2.55,-2.2)) ;
#23447=CARTESIAN_POINT('Origin',(-24.85,2.3,-2.2)) ;
#23448=CARTESIAN_POINT('Origin',(-24.3348780407187,2.05,-1.23015433371742)) ;
#23449=CARTESIAN_POINT('',(-24.0851331751542,2.05,-1.16439100420103)) ;
#23450=CARTESIAN_POINT('',(-24.3202472760712,2.05,-1.487997801951)) ;
#23451=CARTESIAN_POINT('Origin',(-23.,2.05,-2.2)) ;
#23452=CARTESIAN_POINT('',(-24.3791243891352,2.05,-0.950793884383935)) ;
#23453=CARTESIAN_POINT('',(-24.2173209902602,2.05,-1.06835093484243)) ;
#23454=CARTESIAN_POINT('',(-24.6142384900521,2.05,-1.27440068213391)) ;
#23455=CARTESIAN_POINT('',(-24.4966814395937,2.05,-1.11259728325892)) ;
#23456=CARTESIAN_POINT('',(-24.4524350911772,2.05,-1.39195773259241)) ;
#23457=CARTESIAN_POINT('Origin',(-24.2173209902602,2.3,-1.06835093484243)) ;
#23458=CARTESIAN_POINT('',(-24.0851331751542,2.55,-1.16439100420103)) ;
#23459=CARTESIAN_POINT('',(-24.0851331751542,2.3,-1.16439100420103)) ;
#23460=CARTESIAN_POINT('',(-24.3791243891352,2.55,-0.950793884383935)) ;
#23461=CARTESIAN_POINT('',(-24.2173209902602,2.55,-1.06835093484243)) ;
#23462=CARTESIAN_POINT('',(-24.3791243891352,2.3,-0.950793884383935)) ;
#23463=CARTESIAN_POINT('Origin',(-24.4524350911772,2.3,-1.39195773259241)) ;
#23464=CARTESIAN_POINT('',(-24.3202472760712,2.55,-1.487997801951)) ;
#23465=CARTESIAN_POINT('',(-24.3202472760712,2.3,-1.487997801951)) ;
#23466=CARTESIAN_POINT('',(-24.6142384900521,2.55,-1.27440068213391)) ;
#23467=CARTESIAN_POINT('',(-24.6142384900521,2.3,-1.27440068213391)) ;
#23468=CARTESIAN_POINT('',(-24.4524350911772,2.55,-1.39195773259241)) ;
#23469=CARTESIAN_POINT('Origin',(-24.3348780407187,2.55,-1.23015433371742)) ;
#23470=CARTESIAN_POINT('Origin',(-23.,2.55,-2.2)) ;
#23471=CARTESIAN_POINT('',(-24.4966814395937,2.55,-1.11259728325892)) ;
#23472=CARTESIAN_POINT('Origin',(-24.4966814395937,2.3,-1.11259728325892)) ;
#23473=CARTESIAN_POINT('Origin',(-23.5098780407187,2.05,-0.630756748112997)) ;
#23474=CARTESIAN_POINT('',(-23.2691754849877,2.05,-0.724349445742112)) ;
#23475=CARTESIAN_POINT('',(-23.6495980915058,2.05,-0.847956243492091)) ;
#23476=CARTESIAN_POINT('Origin',(-23.,2.05,-2.2)) ;
#23477=CARTESIAN_POINT('',(-23.3814701363346,2.05,-0.378742045978976)) ;
#23478=CARTESIAN_POINT('',(-23.3196667374596,2.05,-0.568953349238007)) ;
#23479=CARTESIAN_POINT('',(-23.7618927428527,2.05,-0.502348843728955)) ;
#23480=CARTESIAN_POINT('',(-23.5716814395937,2.05,-0.440545444853966)) ;
#23481=CARTESIAN_POINT('',(-23.7000893439777,2.05,-0.692560146987986)) ;
#23482=CARTESIAN_POINT('Origin',(-23.3196667374596,2.3,-0.568953349238007)) ;
#23483=CARTESIAN_POINT('',(-23.2691754849877,2.55,-0.724349445742112)) ;
#23484=CARTESIAN_POINT('',(-23.2691754849877,2.3,-0.724349445742112)) ;
#23485=CARTESIAN_POINT('',(-23.3814701363346,2.55,-0.378742045978976)) ;
#23486=CARTESIAN_POINT('',(-23.3196667374596,2.55,-0.568953349238007)) ;
#23487=CARTESIAN_POINT('',(-23.3814701363346,2.3,-0.378742045978976)) ;
#23488=CARTESIAN_POINT('Origin',(-23.7000893439777,2.3,-0.692560146987986)) ;
#23489=CARTESIAN_POINT('',(-23.6495980915058,2.55,-0.847956243492091)) ;
#23490=CARTESIAN_POINT('',(-23.6495980915058,2.3,-0.847956243492091)) ;
#23491=CARTESIAN_POINT('',(-23.7618927428527,2.55,-0.502348843728955)) ;
#23492=CARTESIAN_POINT('',(-23.7618927428527,2.3,-0.502348843728955)) ;
#23493=CARTESIAN_POINT('',(-23.7000893439777,2.55,-0.692560146987986)) ;
#23494=CARTESIAN_POINT('Origin',(-23.5098780407187,2.55,-0.630756748112997)) ;
#23495=CARTESIAN_POINT('Origin',(-23.,2.55,-2.2)) ;
#23496=CARTESIAN_POINT('',(-23.5716814395937,2.55,-0.440545444853966)) ;
#23497=CARTESIAN_POINT('Origin',(-23.5716814395937,2.3,-0.440545444853966)) ;
#23498=CARTESIAN_POINT('Origin',(-22.4901219592813,2.05,-0.630756748112997)) ;
#23499=CARTESIAN_POINT('',(-22.3504019084942,2.05,-0.847956243492089)) ;
#23500=CARTESIAN_POINT('',(-22.7308245150123,2.05,-0.724349445742111)) ;
#23501=CARTESIAN_POINT('Origin',(-23.,2.05,-2.2)) ;
#23502=CARTESIAN_POINT('',(-22.2381072571473,2.05,-0.502348843728955)) ;
#23503=CARTESIAN_POINT('',(-22.2999106560223,2.05,-0.692560146987986)) ;
#23504=CARTESIAN_POINT('',(-22.6185298636654,2.05,-0.378742045978977)) ;
#23505=CARTESIAN_POINT('',(-22.4283185604063,2.05,-0.440545444853966)) ;
#23506=CARTESIAN_POINT('',(-22.6803332625404,2.05,-0.568953349238007)) ;
#23507=CARTESIAN_POINT('Origin',(-22.2999106560223,2.3,-0.692560146987986)) ;
#23508=CARTESIAN_POINT('',(-22.3504019084942,2.55,-0.847956243492089)) ;
#23509=CARTESIAN_POINT('',(-22.3504019084942,2.3,-0.84795624349209)) ;
#23510=CARTESIAN_POINT('',(-22.2381072571473,2.55,-0.502348843728955)) ;
#23511=CARTESIAN_POINT('',(-22.2999106560223,2.55,-0.692560146987986)) ;
#23512=CARTESIAN_POINT('',(-22.2381072571473,2.3,-0.502348843728955)) ;
#23513=CARTESIAN_POINT('Origin',(-22.6803332625404,2.3,-0.568953349238007)) ;
#23514=CARTESIAN_POINT('',(-22.7308245150123,2.55,-0.724349445742111)) ;
#23515=CARTESIAN_POINT('',(-22.7308245150123,2.3,-0.724349445742111)) ;
#23516=CARTESIAN_POINT('',(-22.6185298636654,2.55,-0.378742045978977)) ;
#23517=CARTESIAN_POINT('',(-22.6185298636654,2.3,-0.378742045978977)) ;
#23518=CARTESIAN_POINT('',(-22.6803332625404,2.55,-0.568953349238007)) ;
#23519=CARTESIAN_POINT('Origin',(-22.4901219592813,2.55,-0.630756748112997)) ;
#23520=CARTESIAN_POINT('Origin',(-23.,2.55,-2.2)) ;
#23521=CARTESIAN_POINT('',(-22.4283185604063,2.55,-0.440545444853966)) ;
#23522=CARTESIAN_POINT('Origin',(-22.4283185604063,2.3,-0.440545444853966)) ;
#23523=CARTESIAN_POINT('Origin',(-21.6651219592813,2.05,-1.23015433371742)) ;
#23524=CARTESIAN_POINT('',(-21.6797527239288,2.05,-1.487997801951)) ;
#23525=CARTESIAN_POINT('',(-21.9148668248458,2.05,-1.16439100420103)) ;
#23526=CARTESIAN_POINT('Origin',(-23.,2.05,-2.2)) ;
#23527=CARTESIAN_POINT('',(-21.3857615099479,2.05,-1.27440068213391)) ;
#23528=CARTESIAN_POINT('',(-21.5475649088228,2.05,-1.39195773259241)) ;
#23529=CARTESIAN_POINT('',(-21.6208756108648,2.05,-0.950793884383935)) ;
#23530=CARTESIAN_POINT('',(-21.5033185604063,2.05,-1.11259728325892)) ;
#23531=CARTESIAN_POINT('',(-21.7826790097398,2.05,-1.06835093484243)) ;
#23532=CARTESIAN_POINT('Origin',(-21.5475649088228,2.3,-1.39195773259241)) ;
#23533=CARTESIAN_POINT('',(-21.6797527239288,2.55,-1.487997801951)) ;
#23534=CARTESIAN_POINT('',(-21.6797527239288,2.3,-1.487997801951)) ;
#23535=CARTESIAN_POINT('',(-21.3857615099479,2.55,-1.27440068213391)) ;
#23536=CARTESIAN_POINT('',(-21.5475649088228,2.55,-1.39195773259241)) ;
#23537=CARTESIAN_POINT('',(-21.3857615099479,2.3,-1.27440068213391)) ;
#23538=CARTESIAN_POINT('Origin',(-21.7826790097398,2.3,-1.06835093484243)) ;
#23539=CARTESIAN_POINT('',(-21.9148668248458,2.55,-1.16439100420103)) ;
#23540=CARTESIAN_POINT('',(-21.9148668248458,2.3,-1.16439100420103)) ;
#23541=CARTESIAN_POINT('',(-21.6208756108648,2.55,-0.950793884383935)) ;
#23542=CARTESIAN_POINT('',(-21.6208756108648,2.3,-0.950793884383935)) ;
#23543=CARTESIAN_POINT('',(-21.7826790097398,2.55,-1.06835093484243)) ;
#23544=CARTESIAN_POINT('Origin',(-21.6651219592813,2.55,-1.23015433371742)) ;
#23545=CARTESIAN_POINT('Origin',(-23.,2.55,-2.2)) ;
#23546=CARTESIAN_POINT('',(-21.5033185604063,2.55,-1.11259728325892)) ;
#23547=CARTESIAN_POINT('Origin',(-21.5033185604063,2.3,-1.11259728325892)) ;
#23548=CARTESIAN_POINT('Origin',(-21.35,2.05,-2.2)) ;
#23549=CARTESIAN_POINT('',(-21.5133931252681,2.05,-2.4)) ;
#23550=CARTESIAN_POINT('',(-21.5133931252681,2.05,-2.)) ;
#23551=CARTESIAN_POINT('Origin',(-23.,2.05,-2.2)) ;
#23552=CARTESIAN_POINT('',(-21.15,2.05,-2.4)) ;
#23553=CARTESIAN_POINT('',(-21.35,2.05,-2.4)) ;
#23554=CARTESIAN_POINT('',(-21.15,2.05,-2.)) ;
#23555=CARTESIAN_POINT('',(-21.15,2.05,-2.2)) ;
#23556=CARTESIAN_POINT('',(-21.35,2.05,-2.)) ;
#23557=CARTESIAN_POINT('Origin',(-21.35,2.3,-2.4)) ;
#23558=CARTESIAN_POINT('',(-21.5133931252681,2.55,-2.4)) ;
#23559=CARTESIAN_POINT('',(-21.5133931252681,2.3,-2.4)) ;
#23560=CARTESIAN_POINT('',(-21.15,2.55,-2.4)) ;
#23561=CARTESIAN_POINT('',(-21.35,2.55,-2.4)) ;
#23562=CARTESIAN_POINT('',(-21.15,2.3,-2.4)) ;
#23563=CARTESIAN_POINT('Origin',(-21.35,2.3,-2.)) ;
#23564=CARTESIAN_POINT('',(-21.5133931252681,2.55,-2.)) ;
#23565=CARTESIAN_POINT('',(-21.5133931252681,2.3,-2.)) ;
#23566=CARTESIAN_POINT('',(-21.15,2.55,-2.)) ;
#23567=CARTESIAN_POINT('',(-21.15,2.3,-2.)) ;
#23568=CARTESIAN_POINT('',(-21.35,2.55,-2.)) ;
#23569=CARTESIAN_POINT('Origin',(-21.35,2.55,-2.2)) ;
#23570=CARTESIAN_POINT('Origin',(-23.,2.55,-2.2)) ;
#23571=CARTESIAN_POINT('',(-21.15,2.55,-2.2)) ;
#23572=CARTESIAN_POINT('Origin',(-21.15,2.3,-2.2)) ;
#23573=CARTESIAN_POINT('Origin',(-23.,2.3,-2.2)) ;
#23574=CARTESIAN_POINT('',(-24.5,2.6,-2.2)) ;
#23575=CARTESIAN_POINT('Origin',(-23.,2.6,-2.2)) ;
#23576=CARTESIAN_POINT('',(-24.5,2.3,-2.2)) ;
#23577=CARTESIAN_POINT('',(-24.5,2.,-2.2)) ;
#23578=CARTESIAN_POINT('',(-24.5,2.3,-2.2)) ;
#23579=CARTESIAN_POINT('Origin',(-23.,2.,-2.2)) ;
#23580=CARTESIAN_POINT('Origin',(-23.,2.,-2.2)) ;
#23581=CARTESIAN_POINT('Origin',(-23.,2.6,-2.2)) ;
#24561=UNCERTAINTY_MEASURE_WITH_UNIT(LENGTH_MEASURE(0.001),#24629,
'DISTANCE_ACCURACY_VALUE',
'Maximum model space distance between geometric entities at asserted c
onnectivities') ;
#24580=UNCERTAINTY_MEASURE_WITH_UNIT(LENGTH_MEASURE(0.001),#24629,
'DISTANCE_ACCURACY_VALUE',
'Maximum model space distance between geometric entities at asserted c
onnectivities') ;
#24609=(
GEOMETRIC_REPRESENTATION_CONTEXT(3)
GLOBAL_UNCERTAINTY_ASSIGNED_CONTEXT((#24561))
GLOBAL_UNIT_ASSIGNED_CONTEXT((#24629,#24631,#24632))
REPRESENTATION_CONTEXT('','3D')
) ;
#24628=(
GEOMETRIC_REPRESENTATION_CONTEXT(3)
GLOBAL_UNCERTAINTY_ASSIGNED_CONTEXT((#24580))
GLOBAL_UNIT_ASSIGNED_CONTEXT((#24629,#24631,#24632))
REPRESENTATION_CONTEXT('','3D')
) ;
#24629=(
LENGTH_UNIT()
NAMED_UNIT(*)
SI_UNIT(.CENTI.,.METRE.)
) ;
#24631=(
NAMED_UNIT(*)
PLANE_ANGLE_UNIT()
SI_UNIT($,.RADIAN.)
) ;
#24632=(
NAMED_UNIT(*)
SI_UNIT($,.STERADIAN.)
SOLID_ANGLE_UNIT()
) ;
#24661=SHAPE_DEFINITION_REPRESENTATION(#24730,#24819) ;
#24730=PRODUCT_DEFINITION_SHAPE('',$,#24867) ;
#24819=SHAPE_REPRESENTATION('',(#15008),#24609) ;
#24838=PRODUCT_DEFINITION_CONTEXT('part definition',#24981,'design') ;
#24867=PRODUCT_DEFINITION('FEED_ROLLER_SPROCKET',
'FEED_ROLLER_SPROCKET',#24914,#24838) ;
#24914=PRODUCT_DEFINITION_FORMATION('',$,#25011) ;
#24981=APPLICATION_CONTEXT(
'Core Data for Automotive Mechanical Design Process') ;
#24982=PRODUCT_CONTEXT('part definition',#24981,'mechanical') ;
#25011=PRODUCT('FEED_ROLLER_SPROCKET','FEED_ROLLER_SPROCKET',$,(#24982)) ;
#25030=PRESENTATION_STYLE_ASSIGNMENT((#25040)) ;
#25040=SURFACE_STYLE_USAGE(.BOTH.,#25050) ;
#25050=SURFACE_SIDE_STYLE('',(#25060)) ;
#25060=SURFACE_STYLE_FILL_AREA(#25070) ;
#25070=FILL_AREA_STYLE('Steel - Satin',(#25080)) ;
#25080=FILL_AREA_STYLE_COLOUR('Steel - Satin',#25090) ;
#25090=COLOUR_RGB('Steel - Satin', 0.66274510, 0.83137255, 0.94901961) ;
ENDSEC;
END-ISO-10303-21;
